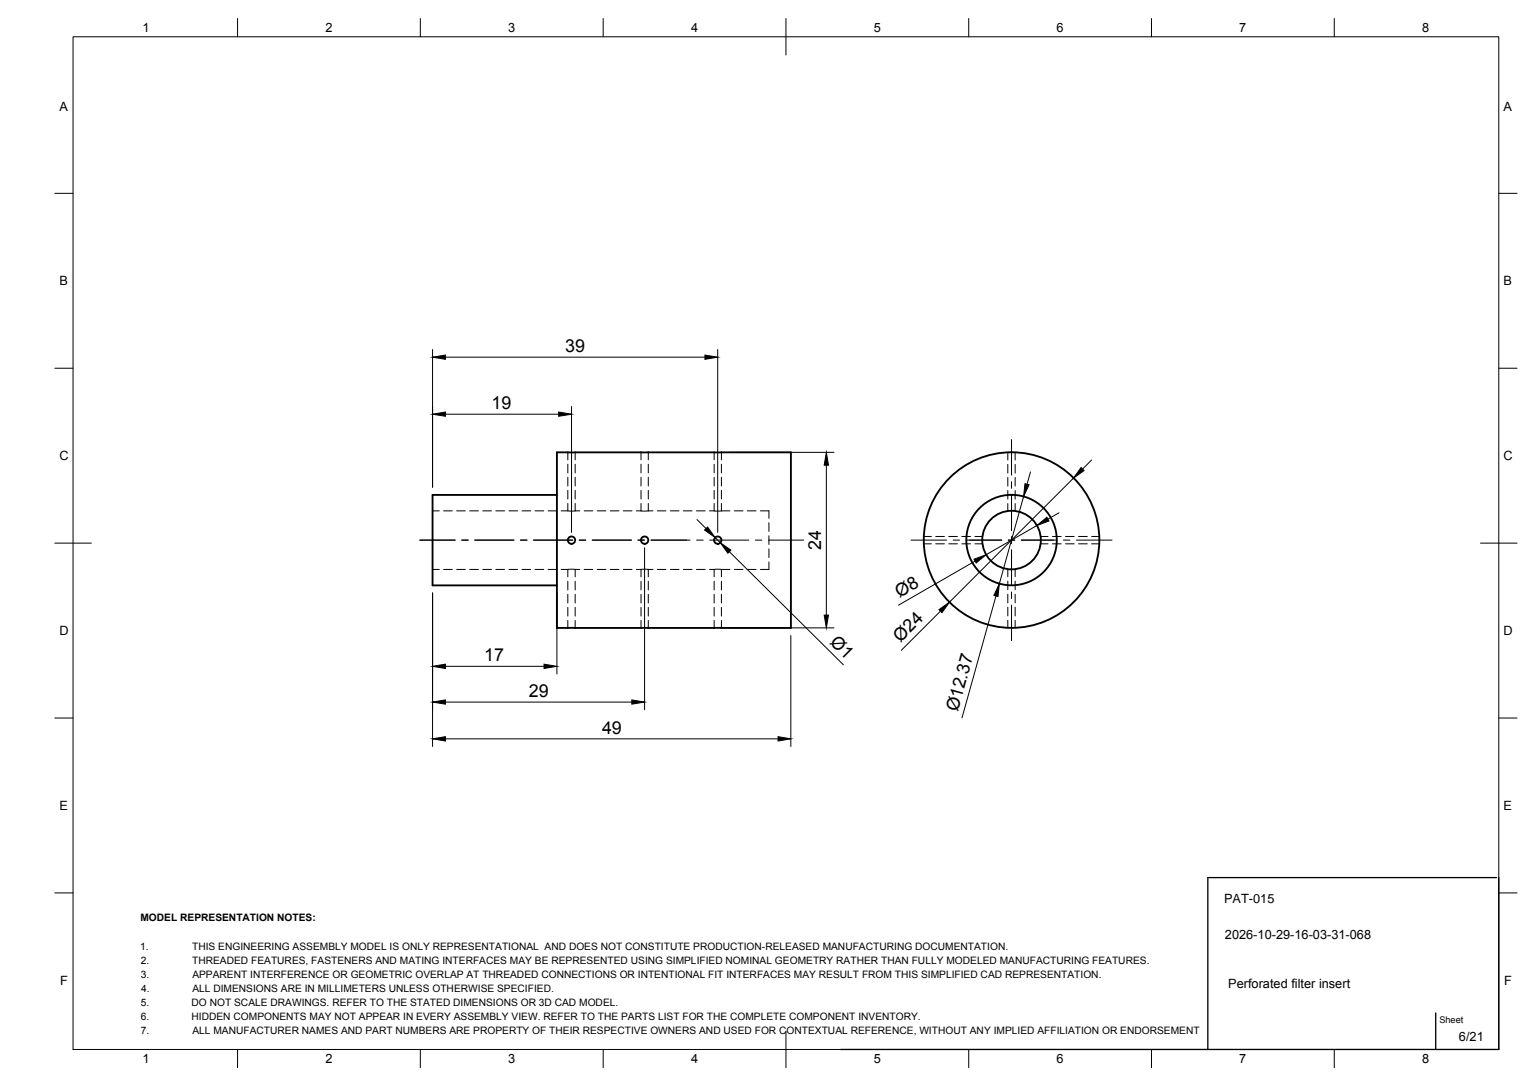
ISO-10303-21;
HEADER;
/* Generated by software containing ST-Developer
 * from STEP Tools, Inc. (www.steptools.com) 
 */

FILE_DESCRIPTION(
/* description */ ('PAT-015'),
/* implementation_level */ '2;1');

FILE_NAME(
/* name */ 'Perforated filter insert.step',
/* time_stamp */ '2026-10-29T16:03:43-07:00',
/* author */ (''),
/* organization */ (''),
/* preprocessor_version */ 'ST-DEVELOPER v20.2',
/* originating_system */ 'Autodesk Translation Framework v15.17.0.0',
/* authorisation */ '');

FILE_SCHEMA (('AUTOMOTIVE_DESIGN { 1 0 10303 214 3 1 1 }'));
ENDSEC;

DATA;
#10=MECHANICAL_DESIGN_GEOMETRIC_PRESENTATION_REPRESENTATION('',(#232),#10266);
#186=SHAPE_REPRESENTATION_RELATIONSHIP('SRR','None',#10357,#209);
#209=ADVANCED_BREP_SHAPE_REPRESENTATION('',(#257),#10245);
#232=STYLED_ITEM('',(#10561),#257);
#257=MANIFOLD_SOLID_BREP('Body1',#4691);
#325=FACE_BOUND('',#967,.T.);
#326=FACE_BOUND('',#968,.T.);
#327=FACE_BOUND('',#969,.T.);
#328=FACE_BOUND('',#970,.T.);
#329=FACE_BOUND('',#971,.T.);
#330=FACE_BOUND('',#972,.T.);
#331=FACE_BOUND('',#973,.T.);
#332=FACE_BOUND('',#974,.T.);
#333=FACE_BOUND('',#975,.T.);
#334=FACE_BOUND('',#979,.T.);
#335=FACE_BOUND('',#981,.T.);
#336=FACE_BOUND('',#982,.T.);
#337=FACE_BOUND('',#983,.T.);
#338=FACE_BOUND('',#984,.T.);
#339=FACE_BOUND('',#985,.T.);
#340=FACE_BOUND('',#986,.T.);
#341=FACE_BOUND('',#987,.T.);
#342=FACE_BOUND('',#988,.T.);
#343=FACE_BOUND('',#989,.T.);
#344=FACE_BOUND('',#991,.T.);
#451=PLANE('',#5134);
#452=PLANE('',#5138);
#453=PLANE('',#5142);
#454=PLANE('',#5143);
#638=FACE_OUTER_BOUND('',#954,.T.);
#639=FACE_OUTER_BOUND('',#955,.T.);
#640=FACE_OUTER_BOUND('',#956,.T.);
#641=FACE_OUTER_BOUND('',#957,.T.);
#642=FACE_OUTER_BOUND('',#958,.T.);
#643=FACE_OUTER_BOUND('',#959,.T.);
#644=FACE_OUTER_BOUND('',#960,.T.);
#645=FACE_OUTER_BOUND('',#961,.T.);
#646=FACE_OUTER_BOUND('',#962,.T.);
#647=FACE_OUTER_BOUND('',#963,.T.);
#648=FACE_OUTER_BOUND('',#964,.T.);
#649=FACE_OUTER_BOUND('',#965,.T.);
#650=FACE_OUTER_BOUND('',#966,.T.);
#651=FACE_OUTER_BOUND('',#976,.T.);
#652=FACE_OUTER_BOUND('',#977,.T.);
#653=FACE_OUTER_BOUND('',#978,.T.);
#654=FACE_OUTER_BOUND('',#980,.T.);
#655=FACE_OUTER_BOUND('',#990,.T.);
#656=FACE_OUTER_BOUND('',#992,.T.);
#954=EDGE_LOOP('',(#3367,#3368,#3369,#3370));
#955=EDGE_LOOP('',(#3371,#3372,#3373,#3374));
#956=EDGE_LOOP('',(#3375,#3376,#3377,#3378));
#957=EDGE_LOOP('',(#3379,#3380,#3381,#3382));
#958=EDGE_LOOP('',(#3383,#3384,#3385,#3386));
#959=EDGE_LOOP('',(#3387,#3388,#3389,#3390));
#960=EDGE_LOOP('',(#3391,#3392,#3393,#3394,#3395,#3396,#3397,#3398));
#961=EDGE_LOOP('',(#3399,#3400,#3401,#3402,#3403,#3404));
#962=EDGE_LOOP('',(#3405,#3406,#3407,#3408,#3409,#3410,#3411,#3412));
#963=EDGE_LOOP('',(#3413,#3414,#3415,#3416,#3417,#3418));
#964=EDGE_LOOP('',(#3419,#3420,#3421,#3422,#3423,#3424,#3425,#3426));
#965=EDGE_LOOP('',(#3427,#3428,#3429,#3430,#3431,#3432));
#966=EDGE_LOOP('',(#3433,#3434,#3435,#3436,#3437,#3438,#3439,#3440,#3441,
#3442,#3443,#3444,#3445,#3446,#3447,#3448,#3449,#3450,#3451));
#967=EDGE_LOOP('',(#3452));
#968=EDGE_LOOP('',(#3453));
#969=EDGE_LOOP('',(#3454));
#970=EDGE_LOOP('',(#3455));
#971=EDGE_LOOP('',(#3456));
#972=EDGE_LOOP('',(#3457));
#973=EDGE_LOOP('',(#3458,#3459));
#974=EDGE_LOOP('',(#3460,#3461));
#975=EDGE_LOOP('',(#3462,#3463));
#976=EDGE_LOOP('',(#3464));
#977=EDGE_LOOP('',(#3465,#3466,#3467,#3468));
#978=EDGE_LOOP('',(#3469));
#979=EDGE_LOOP('',(#3470));
#980=EDGE_LOOP('',(#3471,#3472,#3473,#3474,#3475,#3476,#3477,#3478,#3479,
#3480,#3481,#3482,#3483,#3484,#3485,#3486,#3487,#3488,#3489));
#981=EDGE_LOOP('',(#3490));
#982=EDGE_LOOP('',(#3491));
#983=EDGE_LOOP('',(#3492));
#984=EDGE_LOOP('',(#3493));
#985=EDGE_LOOP('',(#3494));
#986=EDGE_LOOP('',(#3495));
#987=EDGE_LOOP('',(#3496,#3497));
#988=EDGE_LOOP('',(#3498,#3499));
#989=EDGE_LOOP('',(#3500,#3501));
#990=EDGE_LOOP('',(#3502));
#991=EDGE_LOOP('',(#3503));
#992=EDGE_LOOP('',(#3504));
#1277=B_SPLINE_CURVE_WITH_KNOTS('',3,(#7517,#7518,#7519,#7520,#7521,#7522,
#7523,#7524,#7525,#7526,#7527,#7528,#7529,#7530,#7531,#7532,#7533,#7534,
#7535,#7536,#7537,#7538,#7539,#7540,#7541,#7542,#7543,#7544,#7545,#7546,
#7547,#7548,#7549,#7550),.UNSPECIFIED.,.T.,.F.,(4,2,2,2,2,2,2,2,2,2,2,2,
2,2,2,2,4),(0.,0.0188366744349197,0.0376733488698393,0.0565100213871705,
0.0753466939045016,0.0941833664218328,0.113020038939164,0.131856713374084,
0.150693387809003,0.169530062243923,0.188366736678843,0.207203409196174,
0.226040081713505,0.244876754230836,0.263713426748167,0.282550101183087,
0.301386775618006),.UNSPECIFIED.);
#1278=B_SPLINE_CURVE_WITH_KNOTS('',3,(#7553,#7554,#7555,#7556,#7557,#7558,
#7559,#7560,#7561,#7562,#7563,#7564,#7565,#7566,#7567,#7568,#7569,#7570,
#7571,#7572,#7573,#7574,#7575,#7576,#7577,#7578,#7579,#7580,#7581,#7582,
#7583,#7584,#7585,#7586),.UNSPECIFIED.,.T.,.F.,(4,2,2,2,2,2,2,2,2,2,2,2,
2,2,2,2,4),(0.,0.0188556028927646,0.0377112057855292,0.0565666511569687,
0.0754220965284081,0.0942775418998475,0.113132987271287,0.131988590164052,
0.150844193056816,0.169699795949581,0.188555398842345,0.207410844213785,
0.226266289585224,0.245121734956664,0.263977180328103,0.282832783220868,
0.301688386113632),.UNSPECIFIED.);
#1279=B_SPLINE_CURVE_WITH_KNOTS('',3,(#7589,#7590,#7591,#7592,#7593,#7594,
#7595,#7596,#7597,#7598,#7599,#7600,#7601,#7602,#7603,#7604,#7605,#7606,
#7607,#7608,#7609,#7610,#7611,#7612,#7613,#7614,#7615,#7616,#7617,#7618,
#7619,#7620,#7621,#7622),.UNSPECIFIED.,.T.,.F.,(4,2,2,2,2,2,2,2,2,2,2,2,
2,2,2,2,4),(0.,0.0188556028927646,0.0377112057855292,0.0565666511569687,
0.0754220965284081,0.0942775418998475,0.113132987271287,0.131988590164052,
0.150844193056816,0.169699795949581,0.188555398842345,0.207410844213785,
0.226266289585224,0.245121734956664,0.263977180328103,0.282832783220868,
0.301688386113632),.UNSPECIFIED.);
#1280=B_SPLINE_CURVE_WITH_KNOTS('',3,(#7625,#7626,#7627,#7628,#7629,#7630,
#7631,#7632,#7633,#7634,#7635,#7636,#7637,#7638,#7639,#7640,#7641,#7642,
#7643,#7644,#7645,#7646,#7647,#7648,#7649,#7650,#7651,#7652,#7653,#7654,
#7655,#7656,#7657,#7658),.UNSPECIFIED.,.T.,.F.,(4,2,2,2,2,2,2,2,2,2,2,2,
2,2,2,2,4),(0.,0.0188366744349197,0.0376733488698393,0.0565100213871705,
0.0753466939045016,0.0941833664218328,0.113020038939164,0.131856713374084,
0.150693387809003,0.169530062243923,0.188366736678843,0.207203409196174,
0.226040081713505,0.244876754230836,0.263713426748167,0.282550101183087,
0.301386775618006),.UNSPECIFIED.);
#1281=B_SPLINE_CURVE_WITH_KNOTS('',3,(#7661,#7662,#7663,#7664,#7665,#7666,
#7667,#7668,#7669,#7670,#7671,#7672,#7673,#7674,#7675,#7676,#7677,#7678,
#7679,#7680,#7681,#7682,#7683,#7684,#7685,#7686,#7687,#7688,#7689,#7690,
#7691,#7692,#7693,#7694),.UNSPECIFIED.,.T.,.F.,(4,2,2,2,2,2,2,2,2,2,2,2,
2,2,2,2,4),(0.,0.0188366744349197,0.0376733488698393,0.0565100213871705,
0.0753466939045016,0.0941833664218328,0.113020038939164,0.131856713374084,
0.150693387809003,0.169530062243923,0.188366736678843,0.207203409196174,
0.226040081713505,0.244876754230836,0.263713426748167,0.282550101183087,
0.301386775618007),.UNSPECIFIED.);
#1282=B_SPLINE_CURVE_WITH_KNOTS('',3,(#7697,#7698,#7699,#7700,#7701,#7702,
#7703,#7704,#7705,#7706,#7707,#7708,#7709,#7710,#7711,#7712,#7713,#7714,
#7715,#7716,#7717,#7718,#7719,#7720,#7721,#7722,#7723,#7724,#7725,#7726,
#7727,#7728,#7729,#7730),.UNSPECIFIED.,.T.,.F.,(4,2,2,2,2,2,2,2,2,2,2,2,
2,2,2,2,4),(0.,0.0188556028927646,0.0377112057855293,0.0565666511569687,
0.0754220965284081,0.0942775418998476,0.113132987271287,0.131988590164052,
0.150844193056816,0.169699795949581,0.188555398842346,0.207410844213785,
0.226266289585224,0.245121734956664,0.263977180328103,0.282832783220868,
0.301688386113632),.UNSPECIFIED.);
#1283=B_SPLINE_CURVE_WITH_KNOTS('',3,(#7733,#7734,#7735,#7736,#7737,#7738,
#7739,#7740,#7741,#7742,#7743,#7744,#7745,#7746,#7747,#7748,#7749,#7750,
#7751,#7752,#7753,#7754,#7755,#7756,#7757,#7758,#7759,#7760,#7761,#7762,
#7763,#7764,#7765,#7766),.UNSPECIFIED.,.T.,.F.,(4,2,2,2,2,2,2,2,2,2,2,2,
2,2,2,2,4),(0.,0.0188556028927646,0.0377112057855292,0.0565666511569687,
0.0754220965284081,0.0942775418998475,0.113132987271287,0.131988590164052,
0.150844193056816,0.169699795949581,0.188555398842345,0.207410844213785,
0.226266289585224,0.245121734956664,0.263977180328103,0.282832783220868,
0.301688386113632),.UNSPECIFIED.);
#1284=B_SPLINE_CURVE_WITH_KNOTS('',3,(#7769,#7770,#7771,#7772,#7773,#7774,
#7775,#7776,#7777,#7778,#7779,#7780,#7781,#7782,#7783,#7784,#7785,#7786,
#7787,#7788,#7789,#7790,#7791,#7792,#7793,#7794,#7795,#7796,#7797,#7798,
#7799,#7800,#7801,#7802),.UNSPECIFIED.,.T.,.F.,(4,2,2,2,2,2,2,2,2,2,2,2,
2,2,2,2,4),(0.,0.0188366744349198,0.0376733488698396,0.0565100213871707,
0.0753466939045018,0.094183366421833,0.113020038939164,0.131856713374084,
0.150693387809003,0.169530062243923,0.188366736678843,0.207203409196174,
0.226040081713505,0.244876754230836,0.263713426748167,0.282550101183087,
0.301386775618007),.UNSPECIFIED.);
#1285=B_SPLINE_CURVE_WITH_KNOTS('',3,(#7805,#7806,#7807,#7808,#7809,#7810,
#7811,#7812,#7813,#7814,#7815,#7816,#7817,#7818,#7819,#7820,#7821,#7822,
#7823,#7824,#7825,#7826,#7827,#7828,#7829,#7830,#7831,#7832,#7833,#7834,
#7835,#7836,#7837,#7838),.UNSPECIFIED.,.T.,.F.,(4,2,2,2,2,2,2,2,2,2,2,2,
2,2,2,2,4),(0.,0.0188366744349197,0.0376733488698393,0.0565100213871705,
0.0753466939045016,0.0941833664218328,0.113020038939164,0.131856713374084,
0.150693387809003,0.169530062243923,0.188366736678842,0.207203409196173,
0.226040081713505,0.244876754230836,0.263713426748167,0.282550101183086,
0.301386775618006),.UNSPECIFIED.);
#1286=B_SPLINE_CURVE_WITH_KNOTS('',3,(#7841,#7842,#7843,#7844,#7845,#7846,
#7847,#7848,#7849,#7850,#7851,#7852,#7853,#7854,#7855,#7856,#7857,#7858,
#7859,#7860,#7861,#7862,#7863,#7864,#7865,#7866,#7867,#7868,#7869,#7870,
#7871,#7872,#7873,#7874),.UNSPECIFIED.,.T.,.F.,(4,2,2,2,2,2,2,2,2,2,2,2,
2,2,2,2,4),(0.,0.0188556028927646,0.0377112057855292,0.0565666511569687,
0.0754220965284081,0.0942775418998475,0.113132987271287,0.131988590164052,
0.150844193056816,0.169699795949581,0.188555398842345,0.207410844213785,
0.226266289585224,0.245121734956664,0.263977180328103,0.282832783220868,
0.301688386113632),.UNSPECIFIED.);
#1287=B_SPLINE_CURVE_WITH_KNOTS('',3,(#7877,#7878,#7879,#7880,#7881,#7882,
#7883,#7884,#7885,#7886,#7887,#7888,#7889,#7890,#7891,#7892,#7893,#7894,
#7895,#7896,#7897,#7898,#7899,#7900,#7901,#7902,#7903,#7904,#7905,#7906,
#7907,#7908,#7909,#7910),.UNSPECIFIED.,.T.,.F.,(4,2,2,2,2,2,2,2,2,2,2,2,
2,2,2,2,4),(0.,0.0188556028927646,0.0377112057855292,0.0565666511569687,
0.0754220965284081,0.0942775418998475,0.113132987271287,0.131988590164052,
0.150844193056816,0.169699795949581,0.188555398842345,0.207410844213785,
0.226266289585224,0.245121734956664,0.263977180328103,0.282832783220868,
0.301688386113632),.UNSPECIFIED.);
#1288=B_SPLINE_CURVE_WITH_KNOTS('',3,(#7913,#7914,#7915,#7916,#7917,#7918,
#7919,#7920,#7921,#7922,#7923,#7924,#7925,#7926,#7927,#7928,#7929,#7930,
#7931,#7932,#7933,#7934,#7935,#7936,#7937,#7938,#7939,#7940,#7941,#7942,
#7943,#7944,#7945,#7946),.UNSPECIFIED.,.T.,.F.,(4,2,2,2,2,2,2,2,2,2,2,2,
2,2,2,2,4),(0.,0.0188366744349194,0.0376733488698389,0.0565100213871701,
0.0753466939045014,0.0941833664218326,0.113020038939164,0.131856713374083,
0.150693387809003,0.169530062243922,0.188366736678842,0.207203409196173,
0.226040081713504,0.244876754230835,0.263713426748167,0.282550101183086,
0.301386775618006),.UNSPECIFIED.);
#1289=B_SPLINE_CURVE_WITH_KNOTS('',3,(#7950,#7951,#7952,#7953,#7954,#7955,
#7956,#7957,#7958,#7959),.UNSPECIFIED.,.F.,.F.,(4,2,2,2,4),(0.,0.0188366744349197,
0.0376733488698393,0.0565100213871704,0.0753466939045014),.UNSPECIFIED.);
#1290=B_SPLINE_CURVE_WITH_KNOTS('',3,(#7961,#7962,#7963,#7964,#7965,#7966,
#7967,#7968,#7969,#7970),.UNSPECIFIED.,.F.,.F.,(4,2,2,2,4),(0.226040081713504,
0.244876754230835,0.263713426748166,0.282550101183086,0.301386775618006),
 .UNSPECIFIED.);
#1291=B_SPLINE_CURVE_WITH_KNOTS('',3,(#7971,#7972,#7973,#7974,#7975,#7976,
#7977,#7978,#7979,#7980,#7981,#7982,#7983,#7984,#7985,#7986,#7987,#7988),
 .UNSPECIFIED.,.F.,.F.,(4,2,2,2,2,2,2,2,4),(0.0753466939045014,0.0941833664218325,
0.113020038939164,0.131856713374083,0.150693387809003,0.169530062243923,
0.188366736678842,0.207203409196173,0.226040081713504),.UNSPECIFIED.);
#1292=B_SPLINE_CURVE_WITH_KNOTS('',3,(#7992,#7993,#7994,#7995,#7996,#7997,
#7998,#7999,#8000,#8001,#8002,#8003,#8004,#8005,#8006,#8007,#8008,#8009),
 .UNSPECIFIED.,.F.,.F.,(4,2,2,2,2,2,2,2,4),(0.0754220965284079,0.0942775418998473,
0.113132987271287,0.131988590164051,0.150844193056816,0.16969979594958,
0.188555398842345,0.207410844213784,0.226266289585224),.UNSPECIFIED.);
#1293=B_SPLINE_CURVE_WITH_KNOTS('',3,(#8011,#8012,#8013,#8014,#8015,#8016,
#8017,#8018,#8019,#8020),.UNSPECIFIED.,.F.,.F.,(4,2,2,2,4),(0.,0.0188556028927646,
0.0377112057855293,0.0565666511569686,0.0754220965284079),.UNSPECIFIED.);
#1294=B_SPLINE_CURVE_WITH_KNOTS('',3,(#8021,#8022,#8023,#8024,#8025,#8026,
#8027,#8028,#8029,#8030),.UNSPECIFIED.,.F.,.F.,(4,2,2,2,4),(0.226266289585224,
0.245121734956663,0.263977180328102,0.282832783220867,0.301688386113632),
 .UNSPECIFIED.);
#1295=B_SPLINE_CURVE_WITH_KNOTS('',3,(#8034,#8035,#8036,#8037,#8038,#8039,
#8040,#8041,#8042,#8043),.UNSPECIFIED.,.F.,.F.,(4,2,2,2,4),(0.,0.0188556028927646,
0.0377112057855293,0.0565666511569686,0.0754220965284079),.UNSPECIFIED.);
#1296=B_SPLINE_CURVE_WITH_KNOTS('',3,(#8044,#8045,#8046,#8047,#8048,#8049,
#8050,#8051,#8052,#8053,#8054,#8055,#8056,#8057,#8058,#8059,#8060,#8061,
#8062,#8063,#8064,#8065,#8066,#8067,#8068,#8069),.UNSPECIFIED.,.F.,.F.,
(4,2,2,2,2,2,2,2,2,2,2,2,4),(0.0754220965284079,0.0942775418998473,0.113132987271287,
0.131988590164051,0.150844193056816,0.16969979594958,0.188555398842345,
0.207410844213784,0.226266289585224,0.245121734956663,0.263977180328102,
0.282832783220867,0.301688386113632),.UNSPECIFIED.);
#1297=B_SPLINE_CURVE_WITH_KNOTS('',3,(#8073,#8074,#8075,#8076,#8077,#8078,
#8079,#8080,#8081,#8082,#8083,#8084,#8085,#8086,#8087,#8088,#8089,#8090,
#8091,#8092,#8093,#8094,#8095,#8096,#8097,#8098),.UNSPECIFIED.,.F.,.F.,
(4,2,2,2,2,2,2,2,2,2,2,2,4),(0.,0.0188366744349197,0.0376733488698393,0.0565100213871704,
0.0753466939045015,0.0941833664218325,0.113020038939164,0.131856713374083,
0.150693387809003,0.169530062243923,0.188366736678842,0.207203409196173,
0.226040081713504),.UNSPECIFIED.);
#1298=B_SPLINE_CURVE_WITH_KNOTS('',3,(#8099,#8100,#8101,#8102,#8103,#8104,
#8105,#8106,#8107,#8108),.UNSPECIFIED.,.F.,.F.,(4,2,2,2,4),(0.226040081713504,
0.244876754230835,0.263713426748167,0.282550101183086,0.301386775618006),
 .UNSPECIFIED.);
#1299=B_SPLINE_CURVE_WITH_KNOTS('',3,(#8112,#8113,#8114,#8115,#8116,#8117,
#8118,#8119,#8120,#8121),.UNSPECIFIED.,.F.,.F.,(4,2,2,2,4),(0.,0.0188366744349197,
0.0376733488698393,0.0565100213871705,0.0753466939045016),.UNSPECIFIED.);
#1300=B_SPLINE_CURVE_WITH_KNOTS('',3,(#8123,#8124,#8125,#8126,#8127,#8128,
#8129,#8130,#8131,#8132),.UNSPECIFIED.,.F.,.F.,(4,2,2,2,4),(0.226040081713505,
0.244876754230836,0.263713426748167,0.282550101183087,0.301386775618007),
 .UNSPECIFIED.);
#1301=B_SPLINE_CURVE_WITH_KNOTS('',3,(#8133,#8134,#8135,#8136,#8137,#8138,
#8139,#8140,#8141,#8142,#8143,#8144,#8145,#8146,#8147,#8148,#8149,#8150),
 .UNSPECIFIED.,.F.,.F.,(4,2,2,2,2,2,2,2,4),(0.0753466939045016,0.0941833664218328,
0.113020038939164,0.131856713374084,0.150693387809003,0.169530062243923,
0.188366736678843,0.207203409196174,0.226040081713505),.UNSPECIFIED.);
#1302=B_SPLINE_CURVE_WITH_KNOTS('',3,(#8154,#8155,#8156,#8157,#8158,#8159,
#8160,#8161,#8162,#8163,#8164,#8165,#8166,#8167,#8168,#8169,#8170,#8171),
 .UNSPECIFIED.,.F.,.F.,(4,2,2,2,2,2,2,2,4),(0.0754220965284082,0.0942775418998476,
0.113132987271287,0.131988590164052,0.150844193056816,0.169699795949581,
0.188555398842346,0.207410844213785,0.226266289585224),.UNSPECIFIED.);
#1303=B_SPLINE_CURVE_WITH_KNOTS('',3,(#8173,#8174,#8175,#8176,#8177,#8178,
#8179,#8180,#8181,#8182),.UNSPECIFIED.,.F.,.F.,(4,2,2,2,4),(0.,0.0188556028927646,
0.0377112057855293,0.0565666511569687,0.0754220965284082),.UNSPECIFIED.);
#1304=B_SPLINE_CURVE_WITH_KNOTS('',3,(#8183,#8184,#8185,#8186,#8187,#8188,
#8189,#8190,#8191,#8192),.UNSPECIFIED.,.F.,.F.,(4,2,2,2,4),(0.226266289585224,
0.245121734956664,0.263977180328103,0.282832783220868,0.301688386113633),
 .UNSPECIFIED.);
#1305=B_SPLINE_CURVE_WITH_KNOTS('',3,(#8196,#8197,#8198,#8199,#8200,#8201,
#8202,#8203,#8204,#8205),.UNSPECIFIED.,.F.,.F.,(4,2,2,2,4),(0.,0.0188556028927646,
0.0377112057855293,0.0565666511569687,0.0754220965284081),.UNSPECIFIED.);
#1306=B_SPLINE_CURVE_WITH_KNOTS('',3,(#8206,#8207,#8208,#8209,#8210,#8211,
#8212,#8213,#8214,#8215,#8216,#8217,#8218,#8219,#8220,#8221,#8222,#8223,
#8224,#8225,#8226,#8227,#8228,#8229,#8230,#8231),.UNSPECIFIED.,.F.,.F.,
(4,2,2,2,2,2,2,2,2,2,2,2,4),(0.0754220965284081,0.0942775418998476,0.113132987271287,
0.131988590164052,0.150844193056816,0.169699795949581,0.188555398842346,
0.207410844213785,0.226266289585224,0.245121734956664,0.263977180328103,
0.282832783220868,0.301688386113633),.UNSPECIFIED.);
#1307=B_SPLINE_CURVE_WITH_KNOTS('',3,(#8235,#8236,#8237,#8238,#8239,#8240,
#8241,#8242,#8243,#8244,#8245,#8246,#8247,#8248,#8249,#8250,#8251,#8252,
#8253,#8254,#8255,#8256,#8257,#8258,#8259,#8260),.UNSPECIFIED.,.F.,.F.,
(4,2,2,2,2,2,2,2,2,2,2,2,4),(0.,0.0188366744349197,0.0376733488698393,0.0565100213871705,
0.0753466939045017,0.0941833664218329,0.113020038939164,0.131856713374084,
0.150693387809003,0.169530062243923,0.188366736678843,0.207203409196174,
0.226040081713505),.UNSPECIFIED.);
#1308=B_SPLINE_CURVE_WITH_KNOTS('',3,(#8261,#8262,#8263,#8264,#8265,#8266,
#8267,#8268,#8269,#8270),.UNSPECIFIED.,.F.,.F.,(4,2,2,2,4),(0.226040081713505,
0.244876754230836,0.263713426748167,0.282550101183087,0.301386775618007),
 .UNSPECIFIED.);
#1309=B_SPLINE_CURVE_WITH_KNOTS('',3,(#8274,#8275,#8276,#8277,#8278,#8279,
#8280,#8281,#8282,#8283),.UNSPECIFIED.,.F.,.F.,(4,2,2,2,4),(0.,0.0188366744349197,
0.0376733488698393,0.0565100213871705,0.0753466939045016),.UNSPECIFIED.);
#1310=B_SPLINE_CURVE_WITH_KNOTS('',3,(#8285,#8286,#8287,#8288,#8289,#8290,
#8291,#8292,#8293,#8294),.UNSPECIFIED.,.F.,.F.,(4,2,2,2,4),(0.226040081713505,
0.244876754230836,0.263713426748167,0.282550101183087,0.301386775618006),
 .UNSPECIFIED.);
#1311=B_SPLINE_CURVE_WITH_KNOTS('',3,(#8295,#8296,#8297,#8298,#8299,#8300,
#8301,#8302,#8303,#8304,#8305,#8306,#8307,#8308,#8309,#8310,#8311,#8312),
 .UNSPECIFIED.,.F.,.F.,(4,2,2,2,2,2,2,2,4),(0.0753466939045016,0.0941833664218328,
0.113020038939164,0.131856713374084,0.150693387809003,0.169530062243923,
0.188366736678842,0.207203409196173,0.226040081713505),.UNSPECIFIED.);
#1312=B_SPLINE_CURVE_WITH_KNOTS('',3,(#8316,#8317,#8318,#8319,#8320,#8321,
#8322,#8323,#8324,#8325,#8326,#8327,#8328,#8329,#8330,#8331,#8332,#8333),
 .UNSPECIFIED.,.F.,.F.,(4,2,2,2,2,2,2,2,4),(0.0754220965284081,0.0942775418998475,
0.113132987271287,0.131988590164052,0.150844193056816,0.169699795949581,
0.188555398842345,0.207410844213785,0.226266289585224),.UNSPECIFIED.);
#1313=B_SPLINE_CURVE_WITH_KNOTS('',3,(#8335,#8336,#8337,#8338,#8339,#8340,
#8341,#8342,#8343,#8344),.UNSPECIFIED.,.F.,.F.,(4,2,2,2,4),(0.,0.0188556028927646,
0.0377112057855293,0.0565666511569687,0.0754220965284081),.UNSPECIFIED.);
#1314=B_SPLINE_CURVE_WITH_KNOTS('',3,(#8345,#8346,#8347,#8348,#8349,#8350,
#8351,#8352,#8353,#8354),.UNSPECIFIED.,.F.,.F.,(4,2,2,2,4),(0.226266289585224,
0.245121734956664,0.263977180328103,0.282832783220868,0.301688386113632),
 .UNSPECIFIED.);
#1315=B_SPLINE_CURVE_WITH_KNOTS('',3,(#8358,#8359,#8360,#8361,#8362,#8363,
#8364,#8365,#8366,#8367),.UNSPECIFIED.,.F.,.F.,(4,2,2,2,4),(0.,0.0188556028927646,
0.0377112057855293,0.0565666511569687,0.0754220965284081),.UNSPECIFIED.);
#1316=B_SPLINE_CURVE_WITH_KNOTS('',3,(#8368,#8369,#8370,#8371,#8372,#8373,
#8374,#8375,#8376,#8377,#8378,#8379,#8380,#8381,#8382,#8383,#8384,#8385,
#8386,#8387,#8388,#8389,#8390,#8391,#8392,#8393),.UNSPECIFIED.,.F.,.F.,
(4,2,2,2,2,2,2,2,2,2,2,2,4),(0.0754220965284081,0.0942775418998476,0.113132987271287,
0.131988590164052,0.150844193056816,0.169699795949581,0.188555398842345,
0.207410844213785,0.226266289585224,0.245121734956664,0.263977180328103,
0.282832783220868,0.301688386113632),.UNSPECIFIED.);
#1317=B_SPLINE_CURVE_WITH_KNOTS('',3,(#8397,#8398,#8399,#8400,#8401,#8402,
#8403,#8404,#8405,#8406,#8407,#8408,#8409,#8410,#8411,#8412,#8413,#8414,
#8415,#8416,#8417,#8418,#8419,#8420,#8421,#8422),.UNSPECIFIED.,.F.,.F.,
(4,2,2,2,2,2,2,2,2,2,2,2,4),(0.,0.0188366744349194,0.0376733488698389,0.0565100213871702,
0.0753466939045014,0.0941833664218327,0.113020038939164,0.131856713374083,
0.150693387809003,0.169530062243922,0.188366736678842,0.207203409196173,
0.226040081713504),.UNSPECIFIED.);
#1318=B_SPLINE_CURVE_WITH_KNOTS('',3,(#8423,#8424,#8425,#8426,#8427,#8428,
#8429,#8430,#8431,#8432),.UNSPECIFIED.,.F.,.F.,(4,2,2,2,4),(0.226040081713504,
0.244876754230836,0.263713426748167,0.282550101183086,0.301386775618006),
 .UNSPECIFIED.);
#1366=LINE('',#7552,#1646);
#1367=LINE('',#7624,#1647);
#1368=LINE('',#7696,#1648);
#1369=LINE('',#7768,#1649);
#1370=LINE('',#7840,#1650);
#1371=LINE('',#7912,#1651);
#1372=LINE('',#7990,#1652);
#1373=LINE('',#8071,#1653);
#1374=LINE('',#8152,#1654);
#1375=LINE('',#8233,#1655);
#1376=LINE('',#8314,#1656);
#1377=LINE('',#8395,#1657);
#1378=LINE('',#8436,#1658);
#1379=LINE('',#8437,#1659);
#1380=LINE('',#8438,#1660);
#1381=LINE('',#8440,#1661);
#1382=LINE('',#8447,#1662);
#1383=LINE('',#8453,#1663);
#1384=LINE('',#8454,#1664);
#1385=LINE('',#8455,#1665);
#1386=LINE('',#8457,#1666);
#1646=VECTOR('',#5899,0.05);
#1647=VECTOR('',#5902,0.05);
#1648=VECTOR('',#5905,0.05);
#1649=VECTOR('',#5908,0.05);
#1650=VECTOR('',#5911,0.05);
#1651=VECTOR('',#5914,0.05);
#1652=VECTOR('',#5917,0.0499999999999998);
#1653=VECTOR('',#5920,0.0499999999999998);
#1654=VECTOR('',#5923,0.05);
#1655=VECTOR('',#5926,0.05);
#1656=VECTOR('',#5929,0.05);
#1657=VECTOR('',#5932,0.05);
#1658=VECTOR('',#5937,0.4);
#1659=VECTOR('',#5938,0.4);
#1660=VECTOR('',#5939,0.4);
#1661=VECTOR('',#5940,0.4);
#1662=VECTOR('',#5949,0.6185);
#1663=VECTOR('',#5958,1.2);
#1664=VECTOR('',#5959,1.2);
#1665=VECTOR('',#5960,1.2);
#1666=VECTOR('',#5961,1.2);
#1947=CIRCLE('',#5132,0.4);
#1948=CIRCLE('',#5133,0.4);
#1949=CIRCLE('',#5136,0.6185);
#1950=CIRCLE('',#5137,0.6185);
#1951=CIRCLE('',#5140,1.2);
#1952=CIRCLE('',#5141,1.2);
#2201=VERTEX_POINT('',#7516);
#2202=VERTEX_POINT('',#7551);
#2203=VERTEX_POINT('',#7588);
#2204=VERTEX_POINT('',#7623);
#2205=VERTEX_POINT('',#7660);
#2206=VERTEX_POINT('',#7695);
#2207=VERTEX_POINT('',#7732);
#2208=VERTEX_POINT('',#7767);
#2209=VERTEX_POINT('',#7804);
#2210=VERTEX_POINT('',#7839);
#2211=VERTEX_POINT('',#7876);
#2212=VERTEX_POINT('',#7911);
#2213=VERTEX_POINT('',#7948);
#2214=VERTEX_POINT('',#7949);
#2215=VERTEX_POINT('',#7960);
#2216=VERTEX_POINT('',#7989);
#2217=VERTEX_POINT('',#7991);
#2218=VERTEX_POINT('',#8010);
#2219=VERTEX_POINT('',#8032);
#2220=VERTEX_POINT('',#8033);
#2221=VERTEX_POINT('',#8070);
#2222=VERTEX_POINT('',#8072);
#2223=VERTEX_POINT('',#8110);
#2224=VERTEX_POINT('',#8111);
#2225=VERTEX_POINT('',#8122);
#2226=VERTEX_POINT('',#8151);
#2227=VERTEX_POINT('',#8153);
#2228=VERTEX_POINT('',#8172);
#2229=VERTEX_POINT('',#8194);
#2230=VERTEX_POINT('',#8195);
#2231=VERTEX_POINT('',#8232);
#2232=VERTEX_POINT('',#8234);
#2233=VERTEX_POINT('',#8272);
#2234=VERTEX_POINT('',#8273);
#2235=VERTEX_POINT('',#8284);
#2236=VERTEX_POINT('',#8313);
#2237=VERTEX_POINT('',#8315);
#2238=VERTEX_POINT('',#8334);
#2239=VERTEX_POINT('',#8356);
#2240=VERTEX_POINT('',#8357);
#2241=VERTEX_POINT('',#8394);
#2242=VERTEX_POINT('',#8396);
#2243=VERTEX_POINT('',#8434);
#2244=VERTEX_POINT('',#8439);
#2245=VERTEX_POINT('',#8444);
#2246=VERTEX_POINT('',#8446);
#2247=VERTEX_POINT('',#8451);
#2248=VERTEX_POINT('',#8456);
#2639=EDGE_CURVE('',#2201,#2201,#1277,.T.);
#2640=EDGE_CURVE('',#2201,#2202,#1366,.T.);
#2641=EDGE_CURVE('',#2202,#2202,#1278,.T.);
#2642=EDGE_CURVE('',#2203,#2203,#1279,.T.);
#2643=EDGE_CURVE('',#2203,#2204,#1367,.T.);
#2644=EDGE_CURVE('',#2204,#2204,#1280,.T.);
#2645=EDGE_CURVE('',#2205,#2205,#1281,.T.);
#2646=EDGE_CURVE('',#2205,#2206,#1368,.T.);
#2647=EDGE_CURVE('',#2206,#2206,#1282,.T.);
#2648=EDGE_CURVE('',#2207,#2207,#1283,.T.);
#2649=EDGE_CURVE('',#2207,#2208,#1369,.T.);
#2650=EDGE_CURVE('',#2208,#2208,#1284,.T.);
#2651=EDGE_CURVE('',#2209,#2209,#1285,.T.);
#2652=EDGE_CURVE('',#2209,#2210,#1370,.T.);
#2653=EDGE_CURVE('',#2210,#2210,#1286,.T.);
#2654=EDGE_CURVE('',#2211,#2211,#1287,.T.);
#2655=EDGE_CURVE('',#2211,#2212,#1371,.T.);
#2656=EDGE_CURVE('',#2212,#2212,#1288,.T.);
#2657=EDGE_CURVE('',#2213,#2214,#1289,.T.);
#2658=EDGE_CURVE('',#2215,#2213,#1290,.T.);
#2659=EDGE_CURVE('',#2214,#2215,#1291,.T.);
#2660=EDGE_CURVE('',#2214,#2216,#1372,.T.);
#2661=EDGE_CURVE('',#2217,#2216,#1292,.T.);
#2662=EDGE_CURVE('',#2218,#2217,#1293,.T.);
#2663=EDGE_CURVE('',#2216,#2218,#1294,.T.);
#2664=EDGE_CURVE('',#2219,#2220,#1295,.T.);
#2665=EDGE_CURVE('',#2220,#2219,#1296,.T.);
#2666=EDGE_CURVE('',#2220,#2221,#1373,.T.);
#2667=EDGE_CURVE('',#2222,#2221,#1297,.T.);
#2668=EDGE_CURVE('',#2221,#2222,#1298,.T.);
#2669=EDGE_CURVE('',#2223,#2224,#1299,.T.);
#2670=EDGE_CURVE('',#2225,#2223,#1300,.T.);
#2671=EDGE_CURVE('',#2224,#2225,#1301,.T.);
#2672=EDGE_CURVE('',#2224,#2226,#1374,.T.);
#2673=EDGE_CURVE('',#2227,#2226,#1302,.T.);
#2674=EDGE_CURVE('',#2228,#2227,#1303,.T.);
#2675=EDGE_CURVE('',#2226,#2228,#1304,.T.);
#2676=EDGE_CURVE('',#2229,#2230,#1305,.T.);
#2677=EDGE_CURVE('',#2230,#2229,#1306,.T.);
#2678=EDGE_CURVE('',#2230,#2231,#1375,.T.);
#2679=EDGE_CURVE('',#2232,#2231,#1307,.T.);
#2680=EDGE_CURVE('',#2231,#2232,#1308,.T.);
#2681=EDGE_CURVE('',#2233,#2234,#1309,.T.);
#2682=EDGE_CURVE('',#2235,#2233,#1310,.T.);
#2683=EDGE_CURVE('',#2234,#2235,#1311,.T.);
#2684=EDGE_CURVE('',#2234,#2236,#1376,.T.);
#2685=EDGE_CURVE('',#2237,#2236,#1312,.T.);
#2686=EDGE_CURVE('',#2238,#2237,#1313,.T.);
#2687=EDGE_CURVE('',#2236,#2238,#1314,.T.);
#2688=EDGE_CURVE('',#2239,#2240,#1315,.T.);
#2689=EDGE_CURVE('',#2240,#2239,#1316,.T.);
#2690=EDGE_CURVE('',#2240,#2241,#1377,.T.);
#2691=EDGE_CURVE('',#2242,#2241,#1317,.T.);
#2692=EDGE_CURVE('',#2241,#2242,#1318,.T.);
#2693=EDGE_CURVE('',#2243,#2243,#1947,.T.);
#2694=EDGE_CURVE('',#2243,#2217,#1378,.T.);
#2695=EDGE_CURVE('',#2216,#2227,#1379,.T.);
#2696=EDGE_CURVE('',#2226,#2237,#1380,.T.);
#2697=EDGE_CURVE('',#2236,#2244,#1381,.T.);
#2698=EDGE_CURVE('',#2244,#2244,#1948,.T.);
#2699=EDGE_CURVE('',#2245,#2245,#1949,.T.);
#2700=EDGE_CURVE('',#2245,#2246,#1382,.T.);
#2701=EDGE_CURVE('',#2246,#2246,#1950,.T.);
#2702=EDGE_CURVE('',#2247,#2247,#1951,.T.);
#2703=EDGE_CURVE('',#2247,#2234,#1383,.T.);
#2704=EDGE_CURVE('',#2235,#2224,#1384,.T.);
#2705=EDGE_CURVE('',#2225,#2214,#1385,.T.);
#2706=EDGE_CURVE('',#2215,#2248,#1386,.T.);
#2707=EDGE_CURVE('',#2248,#2248,#1952,.T.);
#3367=ORIENTED_EDGE('',*,*,#2639,.F.);
#3368=ORIENTED_EDGE('',*,*,#2640,.T.);
#3369=ORIENTED_EDGE('',*,*,#2641,.F.);
#3370=ORIENTED_EDGE('',*,*,#2640,.F.);
#3371=ORIENTED_EDGE('',*,*,#2642,.F.);
#3372=ORIENTED_EDGE('',*,*,#2643,.T.);
#3373=ORIENTED_EDGE('',*,*,#2644,.F.);
#3374=ORIENTED_EDGE('',*,*,#2643,.F.);
#3375=ORIENTED_EDGE('',*,*,#2645,.F.);
#3376=ORIENTED_EDGE('',*,*,#2646,.T.);
#3377=ORIENTED_EDGE('',*,*,#2647,.F.);
#3378=ORIENTED_EDGE('',*,*,#2646,.F.);
#3379=ORIENTED_EDGE('',*,*,#2648,.F.);
#3380=ORIENTED_EDGE('',*,*,#2649,.T.);
#3381=ORIENTED_EDGE('',*,*,#2650,.F.);
#3382=ORIENTED_EDGE('',*,*,#2649,.F.);
#3383=ORIENTED_EDGE('',*,*,#2651,.F.);
#3384=ORIENTED_EDGE('',*,*,#2652,.T.);
#3385=ORIENTED_EDGE('',*,*,#2653,.F.);
#3386=ORIENTED_EDGE('',*,*,#2652,.F.);
#3387=ORIENTED_EDGE('',*,*,#2654,.F.);
#3388=ORIENTED_EDGE('',*,*,#2655,.T.);
#3389=ORIENTED_EDGE('',*,*,#2656,.F.);
#3390=ORIENTED_EDGE('',*,*,#2655,.F.);
#3391=ORIENTED_EDGE('',*,*,#2657,.F.);
#3392=ORIENTED_EDGE('',*,*,#2658,.F.);
#3393=ORIENTED_EDGE('',*,*,#2659,.F.);
#3394=ORIENTED_EDGE('',*,*,#2660,.T.);
#3395=ORIENTED_EDGE('',*,*,#2661,.F.);
#3396=ORIENTED_EDGE('',*,*,#2662,.F.);
#3397=ORIENTED_EDGE('',*,*,#2663,.F.);
#3398=ORIENTED_EDGE('',*,*,#2660,.F.);
#3399=ORIENTED_EDGE('',*,*,#2664,.F.);
#3400=ORIENTED_EDGE('',*,*,#2665,.F.);
#3401=ORIENTED_EDGE('',*,*,#2666,.T.);
#3402=ORIENTED_EDGE('',*,*,#2667,.F.);
#3403=ORIENTED_EDGE('',*,*,#2668,.F.);
#3404=ORIENTED_EDGE('',*,*,#2666,.F.);
#3405=ORIENTED_EDGE('',*,*,#2669,.F.);
#3406=ORIENTED_EDGE('',*,*,#2670,.F.);
#3407=ORIENTED_EDGE('',*,*,#2671,.F.);
#3408=ORIENTED_EDGE('',*,*,#2672,.T.);
#3409=ORIENTED_EDGE('',*,*,#2673,.F.);
#3410=ORIENTED_EDGE('',*,*,#2674,.F.);
#3411=ORIENTED_EDGE('',*,*,#2675,.F.);
#3412=ORIENTED_EDGE('',*,*,#2672,.F.);
#3413=ORIENTED_EDGE('',*,*,#2676,.F.);
#3414=ORIENTED_EDGE('',*,*,#2677,.F.);
#3415=ORIENTED_EDGE('',*,*,#2678,.T.);
#3416=ORIENTED_EDGE('',*,*,#2679,.F.);
#3417=ORIENTED_EDGE('',*,*,#2680,.F.);
#3418=ORIENTED_EDGE('',*,*,#2678,.F.);
#3419=ORIENTED_EDGE('',*,*,#2681,.F.);
#3420=ORIENTED_EDGE('',*,*,#2682,.F.);
#3421=ORIENTED_EDGE('',*,*,#2683,.F.);
#3422=ORIENTED_EDGE('',*,*,#2684,.T.);
#3423=ORIENTED_EDGE('',*,*,#2685,.F.);
#3424=ORIENTED_EDGE('',*,*,#2686,.F.);
#3425=ORIENTED_EDGE('',*,*,#2687,.F.);
#3426=ORIENTED_EDGE('',*,*,#2684,.F.);
#3427=ORIENTED_EDGE('',*,*,#2688,.F.);
#3428=ORIENTED_EDGE('',*,*,#2689,.F.);
#3429=ORIENTED_EDGE('',*,*,#2690,.T.);
#3430=ORIENTED_EDGE('',*,*,#2691,.F.);
#3431=ORIENTED_EDGE('',*,*,#2692,.F.);
#3432=ORIENTED_EDGE('',*,*,#2690,.F.);
#3433=ORIENTED_EDGE('',*,*,#2693,.F.);
#3434=ORIENTED_EDGE('',*,*,#2694,.T.);
#3435=ORIENTED_EDGE('',*,*,#2661,.T.);
#3436=ORIENTED_EDGE('',*,*,#2695,.T.);
#3437=ORIENTED_EDGE('',*,*,#2673,.T.);
#3438=ORIENTED_EDGE('',*,*,#2696,.T.);
#3439=ORIENTED_EDGE('',*,*,#2685,.T.);
#3440=ORIENTED_EDGE('',*,*,#2697,.T.);
#3441=ORIENTED_EDGE('',*,*,#2698,.F.);
#3442=ORIENTED_EDGE('',*,*,#2697,.F.);
#3443=ORIENTED_EDGE('',*,*,#2687,.T.);
#3444=ORIENTED_EDGE('',*,*,#2686,.T.);
#3445=ORIENTED_EDGE('',*,*,#2696,.F.);
#3446=ORIENTED_EDGE('',*,*,#2675,.T.);
#3447=ORIENTED_EDGE('',*,*,#2674,.T.);
#3448=ORIENTED_EDGE('',*,*,#2695,.F.);
#3449=ORIENTED_EDGE('',*,*,#2663,.T.);
#3450=ORIENTED_EDGE('',*,*,#2662,.T.);
#3451=ORIENTED_EDGE('',*,*,#2694,.F.);
#3452=ORIENTED_EDGE('',*,*,#2642,.T.);
#3453=ORIENTED_EDGE('',*,*,#2641,.T.);
#3454=ORIENTED_EDGE('',*,*,#2648,.T.);
#3455=ORIENTED_EDGE('',*,*,#2647,.T.);
#3456=ORIENTED_EDGE('',*,*,#2654,.T.);
#3457=ORIENTED_EDGE('',*,*,#2653,.T.);
#3458=ORIENTED_EDGE('',*,*,#2664,.T.);
#3459=ORIENTED_EDGE('',*,*,#2665,.T.);
#3460=ORIENTED_EDGE('',*,*,#2676,.T.);
#3461=ORIENTED_EDGE('',*,*,#2677,.T.);
#3462=ORIENTED_EDGE('',*,*,#2688,.T.);
#3463=ORIENTED_EDGE('',*,*,#2689,.T.);
#3464=ORIENTED_EDGE('',*,*,#2693,.T.);
#3465=ORIENTED_EDGE('',*,*,#2699,.F.);
#3466=ORIENTED_EDGE('',*,*,#2700,.T.);
#3467=ORIENTED_EDGE('',*,*,#2701,.F.);
#3468=ORIENTED_EDGE('',*,*,#2700,.F.);
#3469=ORIENTED_EDGE('',*,*,#2699,.T.);
#3470=ORIENTED_EDGE('',*,*,#2698,.T.);
#3471=ORIENTED_EDGE('',*,*,#2702,.F.);
#3472=ORIENTED_EDGE('',*,*,#2703,.T.);
#3473=ORIENTED_EDGE('',*,*,#2683,.T.);
#3474=ORIENTED_EDGE('',*,*,#2704,.T.);
#3475=ORIENTED_EDGE('',*,*,#2671,.T.);
#3476=ORIENTED_EDGE('',*,*,#2705,.T.);
#3477=ORIENTED_EDGE('',*,*,#2659,.T.);
#3478=ORIENTED_EDGE('',*,*,#2706,.T.);
#3479=ORIENTED_EDGE('',*,*,#2707,.T.);
#3480=ORIENTED_EDGE('',*,*,#2706,.F.);
#3481=ORIENTED_EDGE('',*,*,#2658,.T.);
#3482=ORIENTED_EDGE('',*,*,#2657,.T.);
#3483=ORIENTED_EDGE('',*,*,#2705,.F.);
#3484=ORIENTED_EDGE('',*,*,#2670,.T.);
#3485=ORIENTED_EDGE('',*,*,#2669,.T.);
#3486=ORIENTED_EDGE('',*,*,#2704,.F.);
#3487=ORIENTED_EDGE('',*,*,#2682,.T.);
#3488=ORIENTED_EDGE('',*,*,#2681,.T.);
#3489=ORIENTED_EDGE('',*,*,#2703,.F.);
#3490=ORIENTED_EDGE('',*,*,#2644,.T.);
#3491=ORIENTED_EDGE('',*,*,#2639,.T.);
#3492=ORIENTED_EDGE('',*,*,#2650,.T.);
#3493=ORIENTED_EDGE('',*,*,#2645,.T.);
#3494=ORIENTED_EDGE('',*,*,#2656,.T.);
#3495=ORIENTED_EDGE('',*,*,#2651,.T.);
#3496=ORIENTED_EDGE('',*,*,#2667,.T.);
#3497=ORIENTED_EDGE('',*,*,#2668,.T.);
#3498=ORIENTED_EDGE('',*,*,#2679,.T.);
#3499=ORIENTED_EDGE('',*,*,#2680,.T.);
#3500=ORIENTED_EDGE('',*,*,#2691,.T.);
#3501=ORIENTED_EDGE('',*,*,#2692,.T.);
#3502=ORIENTED_EDGE('',*,*,#2702,.T.);
#3503=ORIENTED_EDGE('',*,*,#2701,.T.);
#3504=ORIENTED_EDGE('',*,*,#2707,.F.);
#4326=CYLINDRICAL_SURFACE('',#5119,0.05);
#4327=CYLINDRICAL_SURFACE('',#5120,0.05);
#4328=CYLINDRICAL_SURFACE('',#5121,0.05);
#4329=CYLINDRICAL_SURFACE('',#5122,0.05);
#4330=CYLINDRICAL_SURFACE('',#5123,0.05);
#4331=CYLINDRICAL_SURFACE('',#5124,0.05);
#4332=CYLINDRICAL_SURFACE('',#5125,0.0499999999999998);
#4333=CYLINDRICAL_SURFACE('',#5126,0.0499999999999998);
#4334=CYLINDRICAL_SURFACE('',#5127,0.05);
#4335=CYLINDRICAL_SURFACE('',#5128,0.05);
#4336=CYLINDRICAL_SURFACE('',#5129,0.05);
#4337=CYLINDRICAL_SURFACE('',#5130,0.05);
#4338=CYLINDRICAL_SURFACE('',#5131,0.4);
#4339=CYLINDRICAL_SURFACE('',#5135,0.6185);
#4340=CYLINDRICAL_SURFACE('',#5139,1.2);
#4473=ADVANCED_FACE('',(#638),#4326,.F.);
#4474=ADVANCED_FACE('',(#639),#4327,.F.);
#4475=ADVANCED_FACE('',(#640),#4328,.F.);
#4476=ADVANCED_FACE('',(#641),#4329,.F.);
#4477=ADVANCED_FACE('',(#642),#4330,.F.);
#4478=ADVANCED_FACE('',(#643),#4331,.F.);
#4479=ADVANCED_FACE('',(#644),#4332,.F.);
#4480=ADVANCED_FACE('',(#645),#4333,.F.);
#4481=ADVANCED_FACE('',(#646),#4334,.F.);
#4482=ADVANCED_FACE('',(#647),#4335,.F.);
#4483=ADVANCED_FACE('',(#648),#4336,.F.);
#4484=ADVANCED_FACE('',(#649),#4337,.F.);
#4485=ADVANCED_FACE('',(#650,#325,#326,#327,#328,#329,#330,#331,#332,#333),
#4338,.F.);
#4486=ADVANCED_FACE('',(#651),#451,.T.);
#4487=ADVANCED_FACE('',(#652),#4339,.T.);
#4488=ADVANCED_FACE('',(#653,#334),#452,.T.);
#4489=ADVANCED_FACE('',(#654,#335,#336,#337,#338,#339,#340,#341,#342,#343),
#4340,.T.);
#4490=ADVANCED_FACE('',(#655,#344),#453,.T.);
#4491=ADVANCED_FACE('',(#656),#454,.F.);
#4691=CLOSED_SHELL('',(#4473,#4474,#4475,#4476,#4477,#4478,#4479,#4480,
#4481,#4482,#4483,#4484,#4485,#4486,#4487,#4488,#4489,#4490,#4491));
#5118=AXIS2_PLACEMENT_3D('',#7514,#5895,#5896);
#5119=AXIS2_PLACEMENT_3D('',#7515,#5897,#5898);
#5120=AXIS2_PLACEMENT_3D('',#7587,#5900,#5901);
#5121=AXIS2_PLACEMENT_3D('',#7659,#5903,#5904);
#5122=AXIS2_PLACEMENT_3D('',#7731,#5906,#5907);
#5123=AXIS2_PLACEMENT_3D('',#7803,#5909,#5910);
#5124=AXIS2_PLACEMENT_3D('',#7875,#5912,#5913);
#5125=AXIS2_PLACEMENT_3D('',#7947,#5915,#5916);
#5126=AXIS2_PLACEMENT_3D('',#8031,#5918,#5919);
#5127=AXIS2_PLACEMENT_3D('',#8109,#5921,#5922);
#5128=AXIS2_PLACEMENT_3D('',#8193,#5924,#5925);
#5129=AXIS2_PLACEMENT_3D('',#8271,#5927,#5928);
#5130=AXIS2_PLACEMENT_3D('',#8355,#5930,#5931);
#5131=AXIS2_PLACEMENT_3D('',#8433,#5933,#5934);
#5132=AXIS2_PLACEMENT_3D('',#8435,#5935,#5936);
#5133=AXIS2_PLACEMENT_3D('',#8441,#5941,#5942);
#5134=AXIS2_PLACEMENT_3D('',#8442,#5943,#5944);
#5135=AXIS2_PLACEMENT_3D('',#8443,#5945,#5946);
#5136=AXIS2_PLACEMENT_3D('',#8445,#5947,#5948);
#5137=AXIS2_PLACEMENT_3D('',#8448,#5950,#5951);
#5138=AXIS2_PLACEMENT_3D('',#8449,#5952,#5953);
#5139=AXIS2_PLACEMENT_3D('',#8450,#5954,#5955);
#5140=AXIS2_PLACEMENT_3D('',#8452,#5956,#5957);
#5141=AXIS2_PLACEMENT_3D('',#8458,#5962,#5963);
#5142=AXIS2_PLACEMENT_3D('',#8459,#5964,#5965);
#5143=AXIS2_PLACEMENT_3D('',#8460,#5966,#5967);
#5895=DIRECTION('axis',(0.,0.,1.));
#5896=DIRECTION('refdir',(1.,0.,0.));
#5897=DIRECTION('center_axis',(0.,1.,0.));
#5898=DIRECTION('ref_axis',(1.,0.,0.));
#5899=DIRECTION('',(0.,1.,0.));
#5900=DIRECTION('center_axis',(0.,1.,0.));
#5901=DIRECTION('ref_axis',(1.,0.,0.));
#5902=DIRECTION('',(0.,1.,0.));
#5903=DIRECTION('center_axis',(0.,1.,0.));
#5904=DIRECTION('ref_axis',(1.,0.,0.));
#5905=DIRECTION('',(0.,1.,0.));
#5906=DIRECTION('center_axis',(0.,1.,0.));
#5907=DIRECTION('ref_axis',(1.,0.,0.));
#5908=DIRECTION('',(0.,1.,0.));
#5909=DIRECTION('center_axis',(0.,1.,0.));
#5910=DIRECTION('ref_axis',(1.,0.,0.));
#5911=DIRECTION('',(0.,1.,0.));
#5912=DIRECTION('center_axis',(0.,1.,0.));
#5913=DIRECTION('ref_axis',(1.,0.,0.));
#5914=DIRECTION('',(0.,1.,0.));
#5915=DIRECTION('center_axis',(1.,0.,0.));
#5916=DIRECTION('ref_axis',(0.,0.,-1.));
#5917=DIRECTION('',(1.,0.,0.));
#5918=DIRECTION('center_axis',(1.,0.,0.));
#5919=DIRECTION('ref_axis',(0.,0.,-1.));
#5920=DIRECTION('',(1.,0.,0.));
#5921=DIRECTION('center_axis',(1.,0.,0.));
#5922=DIRECTION('ref_axis',(0.,0.,-1.));
#5923=DIRECTION('',(1.,0.,0.));
#5924=DIRECTION('center_axis',(1.,0.,0.));
#5925=DIRECTION('ref_axis',(0.,0.,-1.));
#5926=DIRECTION('',(1.,0.,0.));
#5927=DIRECTION('center_axis',(1.,0.,0.));
#5928=DIRECTION('ref_axis',(0.,0.,-1.));
#5929=DIRECTION('',(1.,0.,0.));
#5930=DIRECTION('center_axis',(1.,0.,0.));
#5931=DIRECTION('ref_axis',(0.,0.,-1.));
#5932=DIRECTION('',(1.,0.,0.));
#5933=DIRECTION('center_axis',(0.,0.,1.));
#5934=DIRECTION('ref_axis',(1.,0.,0.));
#5935=DIRECTION('center_axis',(0.,0.,1.));
#5936=DIRECTION('ref_axis',(1.,0.,0.));
#5937=DIRECTION('',(0.,0.,1.));
#5938=DIRECTION('',(0.,0.,1.));
#5939=DIRECTION('',(0.,0.,1.));
#5940=DIRECTION('',(0.,0.,1.));
#5941=DIRECTION('center_axis',(0.,0.,-1.));
#5942=DIRECTION('ref_axis',(1.,0.,0.));
#5943=DIRECTION('center_axis',(0.,0.,1.));
#5944=DIRECTION('ref_axis',(1.,0.,0.));
#5945=DIRECTION('center_axis',(0.,0.,1.));
#5946=DIRECTION('ref_axis',(1.,0.,0.));
#5947=DIRECTION('center_axis',(0.,0.,1.));
#5948=DIRECTION('ref_axis',(1.,0.,0.));
#5949=DIRECTION('',(0.,0.,-1.));
#5950=DIRECTION('center_axis',(0.,0.,-1.));
#5951=DIRECTION('ref_axis',(1.,0.,0.));
#5952=DIRECTION('center_axis',(0.,0.,1.));
#5953=DIRECTION('ref_axis',(1.,0.,0.));
#5954=DIRECTION('center_axis',(0.,0.,1.));
#5955=DIRECTION('ref_axis',(1.,0.,0.));
#5956=DIRECTION('center_axis',(0.,0.,1.));
#5957=DIRECTION('ref_axis',(1.,0.,0.));
#5958=DIRECTION('',(0.,0.,-1.));
#5959=DIRECTION('',(0.,0.,-1.));
#5960=DIRECTION('',(0.,0.,-1.));
#5961=DIRECTION('',(0.,0.,-1.));
#5962=DIRECTION('center_axis',(0.,0.,1.));
#5963=DIRECTION('ref_axis',(1.,0.,0.));
#5964=DIRECTION('center_axis',(0.,0.,1.));
#5965=DIRECTION('ref_axis',(1.,0.,0.));
#5966=DIRECTION('center_axis',(0.,0.,1.));
#5967=DIRECTION('ref_axis',(1.,0.,0.));
#7514=CARTESIAN_POINT('',(0.,0.,0.));
#7515=CARTESIAN_POINT('Origin',(0.,-1.3,-2.5));
#7516=CARTESIAN_POINT('',(-0.05,-1.19895788082818,-2.5));
#7517=CARTESIAN_POINT('Ctrl Pts',(-0.05,-1.19895788082818,-2.5));
#7518=CARTESIAN_POINT('Ctrl Pts',(-0.05,-1.19895788082818,-2.49372110852169));
#7519=CARTESIAN_POINT('Ctrl Pts',(-0.0487450133099081,-1.19901227819454,
-2.48702419537593));
#7520=CARTESIAN_POINT('Ctrl Pts',(-0.0436421041657014,-1.19920885850753,
-2.47470544370928));
#7521=CARTESIAN_POINT('Ctrl Pts',(-0.0397942217705328,-1.1993482149535,
-2.46908354365188));
#7522=CARTESIAN_POINT('Ctrl Pts',(-0.0309164568000038,-1.19960989221221,
-2.46020577868135));
#7523=CARTESIAN_POINT('Ctrl Pts',(-0.0252945565319674,-1.19974919586288,
-2.45635789595805));
#7524=CARTESIAN_POINT('Ctrl Pts',(-0.0129758042228731,-1.19994565546462,
-2.45125498650009));
#7525=CARTESIAN_POINT('Ctrl Pts',(-0.00627889083911039,-1.2,-2.45));
#7526=CARTESIAN_POINT('Ctrl Pts',(0.00627889083911038,-1.2,-2.45));
#7527=CARTESIAN_POINT('Ctrl Pts',(0.012975804222873,-1.19994565546462,-2.45125498650009));
#7528=CARTESIAN_POINT('Ctrl Pts',(0.0252945565319674,-1.19974919586288,
-2.45635789595805));
#7529=CARTESIAN_POINT('Ctrl Pts',(0.0309164568000038,-1.19960989221221,
-2.46020577868135));
#7530=CARTESIAN_POINT('Ctrl Pts',(0.0397942217705328,-1.1993482149535,-2.46908354365188));
#7531=CARTESIAN_POINT('Ctrl Pts',(0.0436421041657014,-1.19920885850753,
-2.47470544370928));
#7532=CARTESIAN_POINT('Ctrl Pts',(0.0487450133099081,-1.19901227819454,
-2.48702419537593));
#7533=CARTESIAN_POINT('Ctrl Pts',(0.05,-1.19895788082818,-2.49372110852169));
#7534=CARTESIAN_POINT('Ctrl Pts',(0.05,-1.19895788082818,-2.50627889147831));
#7535=CARTESIAN_POINT('Ctrl Pts',(0.0487450133099081,-1.19901227819454,
-2.51297580462407));
#7536=CARTESIAN_POINT('Ctrl Pts',(0.0436421041657014,-1.19920885850753,
-2.52529455629072));
#7537=CARTESIAN_POINT('Ctrl Pts',(0.0397942217705328,-1.1993482149535,-2.53091645634812));
#7538=CARTESIAN_POINT('Ctrl Pts',(0.0309164568000038,-1.19960989221221,
-2.53979422131865));
#7539=CARTESIAN_POINT('Ctrl Pts',(0.0252945565319675,-1.19974919586288,
-2.54364210404195));
#7540=CARTESIAN_POINT('Ctrl Pts',(0.0129758042228731,-1.19994565546462,
-2.54874501349991));
#7541=CARTESIAN_POINT('Ctrl Pts',(0.0062788908391104,-1.2,-2.55));
#7542=CARTESIAN_POINT('Ctrl Pts',(-0.00627889083911037,-1.2,-2.55));
#7543=CARTESIAN_POINT('Ctrl Pts',(-0.012975804222873,-1.19994565546462,
-2.54874501349991));
#7544=CARTESIAN_POINT('Ctrl Pts',(-0.0252945565319674,-1.19974919586288,
-2.54364210404195));
#7545=CARTESIAN_POINT('Ctrl Pts',(-0.0309164568000038,-1.19960989221221,
-2.53979422131865));
#7546=CARTESIAN_POINT('Ctrl Pts',(-0.0397942217705328,-1.1993482149535,
-2.53091645634812));
#7547=CARTESIAN_POINT('Ctrl Pts',(-0.0436421041657014,-1.19920885850753,
-2.52529455629072));
#7548=CARTESIAN_POINT('Ctrl Pts',(-0.0487450133099081,-1.19901227819454,
-2.51297580462407));
#7549=CARTESIAN_POINT('Ctrl Pts',(-0.05,-1.19895788082818,-2.50627889147831));
#7550=CARTESIAN_POINT('Ctrl Pts',(-0.05,-1.19895788082818,-2.5));
#7551=CARTESIAN_POINT('',(-0.05,-0.396862696659689,-2.5));
#7552=CARTESIAN_POINT('',(-0.05,-1.3,-2.5));
#7553=CARTESIAN_POINT('Ctrl Pts',(-0.05,-0.396862696659689,-2.5));
#7554=CARTESIAN_POINT('Ctrl Pts',(-0.05,-0.396862696659689,-2.50628520096426));
#7555=CARTESIAN_POINT('Ctrl Pts',(-0.0487425534891116,-0.397027412247524,
-2.51298480122901));
#7556=CARTESIAN_POINT('Ctrl Pts',(-0.0436378373878618,-0.397620851691571,
-2.52530179409386));
#7557=CARTESIAN_POINT('Ctrl Pts',(-0.0397909243921696,-0.398040841710914,
-2.53091975372649));
#7558=CARTESIAN_POINT('Ctrl Pts',(-0.0309197907817458,-0.398828027526425,
-2.53979088733691));
#7559=CARTESIAN_POINT('Ctrl Pts',(-0.0253018150396577,-0.399246581249293,
-2.5436378293633));
#7560=CARTESIAN_POINT('Ctrl Pts',(-0.0129847676279313,-0.399836729543542,
-2.5487425667586));
#7561=CARTESIAN_POINT('Ctrl Pts',(-0.00628514845714647,-0.4,-2.55));
#7562=CARTESIAN_POINT('Ctrl Pts',(0.00628514845714648,-0.4,-2.55));
#7563=CARTESIAN_POINT('Ctrl Pts',(0.012984767627931,-0.399836729543542,
-2.5487425667586));
#7564=CARTESIAN_POINT('Ctrl Pts',(0.0253018150396574,-0.399246581249293,
-2.5436378293633));
#7565=CARTESIAN_POINT('Ctrl Pts',(0.0309197907817458,-0.398828027526425,
-2.53979088733691));
#7566=CARTESIAN_POINT('Ctrl Pts',(0.0397909243921696,-0.398040841710914,
-2.53091975372649));
#7567=CARTESIAN_POINT('Ctrl Pts',(0.0436378373878616,-0.397620851691571,
-2.52530179409386));
#7568=CARTESIAN_POINT('Ctrl Pts',(0.0487425534891115,-0.397027412247524,
-2.51298480122901));
#7569=CARTESIAN_POINT('Ctrl Pts',(0.05,-0.396862696659689,-2.50628520096426));
#7570=CARTESIAN_POINT('Ctrl Pts',(0.05,-0.396862696659689,-2.49371479903574));
#7571=CARTESIAN_POINT('Ctrl Pts',(0.0487425534891116,-0.397027412247524,
-2.48701519877099));
#7572=CARTESIAN_POINT('Ctrl Pts',(0.0436378373878618,-0.397620851691571,
-2.47469820590614));
#7573=CARTESIAN_POINT('Ctrl Pts',(0.0397909243921696,-0.398040841710914,
-2.46908024627351));
#7574=CARTESIAN_POINT('Ctrl Pts',(0.0309197907817458,-0.398828027526425,
-2.46020911266309));
#7575=CARTESIAN_POINT('Ctrl Pts',(0.0253018150396577,-0.399246581249293,
-2.4563621706367));
#7576=CARTESIAN_POINT('Ctrl Pts',(0.0129847676279313,-0.399836729543542,
-2.4512574332414));
#7577=CARTESIAN_POINT('Ctrl Pts',(0.00628514845714648,-0.4,-2.45));
#7578=CARTESIAN_POINT('Ctrl Pts',(-0.00628514845714647,-0.4,-2.45));
#7579=CARTESIAN_POINT('Ctrl Pts',(-0.0129847676279313,-0.399836729543542,
-2.4512574332414));
#7580=CARTESIAN_POINT('Ctrl Pts',(-0.0253018150396577,-0.399246581249293,
-2.4563621706367));
#7581=CARTESIAN_POINT('Ctrl Pts',(-0.0309197907817458,-0.398828027526425,
-2.46020911266309));
#7582=CARTESIAN_POINT('Ctrl Pts',(-0.0397909243921696,-0.398040841710914,
-2.46908024627351));
#7583=CARTESIAN_POINT('Ctrl Pts',(-0.0436378373878618,-0.397620851691571,
-2.47469820590614));
#7584=CARTESIAN_POINT('Ctrl Pts',(-0.0487425534891116,-0.397027412247524,
-2.48701519877099));
#7585=CARTESIAN_POINT('Ctrl Pts',(-0.05,-0.396862696659689,-2.49371479903574));
#7586=CARTESIAN_POINT('Ctrl Pts',(-0.05,-0.396862696659689,-2.5));
#7587=CARTESIAN_POINT('Origin',(0.,-1.3,-2.5));
#7588=CARTESIAN_POINT('',(-0.05,0.396862696659689,-2.5));
#7589=CARTESIAN_POINT('Ctrl Pts',(-0.05,0.396862696659689,-2.5));
#7590=CARTESIAN_POINT('Ctrl Pts',(-0.05,0.396862696659689,-2.49371479903574));
#7591=CARTESIAN_POINT('Ctrl Pts',(-0.0487425534891116,0.397027412247524,
-2.48701519877099));
#7592=CARTESIAN_POINT('Ctrl Pts',(-0.0436378373878618,0.397620851691571,
-2.47469820590614));
#7593=CARTESIAN_POINT('Ctrl Pts',(-0.0397909243921696,0.398040841710914,
-2.46908024627351));
#7594=CARTESIAN_POINT('Ctrl Pts',(-0.0309197907817458,0.398828027526425,
-2.46020911266309));
#7595=CARTESIAN_POINT('Ctrl Pts',(-0.0253018150396577,0.399246581249293,
-2.4563621706367));
#7596=CARTESIAN_POINT('Ctrl Pts',(-0.0129847676279313,0.399836729543542,
-2.4512574332414));
#7597=CARTESIAN_POINT('Ctrl Pts',(-0.00628514845714647,0.4,-2.45));
#7598=CARTESIAN_POINT('Ctrl Pts',(0.00628514845714648,0.4,-2.45));
#7599=CARTESIAN_POINT('Ctrl Pts',(0.0129847676279313,0.399836729543542,
-2.4512574332414));
#7600=CARTESIAN_POINT('Ctrl Pts',(0.0253018150396577,0.399246581249293,
-2.4563621706367));
#7601=CARTESIAN_POINT('Ctrl Pts',(0.0309197907817458,0.398828027526425,
-2.46020911266309));
#7602=CARTESIAN_POINT('Ctrl Pts',(0.0397909243921696,0.398040841710914,
-2.46908024627351));
#7603=CARTESIAN_POINT('Ctrl Pts',(0.0436378373878621,0.397620851691571,
-2.47469820590614));
#7604=CARTESIAN_POINT('Ctrl Pts',(0.0487425534891117,0.397027412247524,
-2.48701519877099));
#7605=CARTESIAN_POINT('Ctrl Pts',(0.05,0.396862696659689,-2.49371479903574));
#7606=CARTESIAN_POINT('Ctrl Pts',(0.05,0.396862696659689,-2.50628520096426));
#7607=CARTESIAN_POINT('Ctrl Pts',(0.0487425534891116,0.397027412247524,
-2.51298480122901));
#7608=CARTESIAN_POINT('Ctrl Pts',(0.0436378373878618,0.397620851691571,
-2.52530179409386));
#7609=CARTESIAN_POINT('Ctrl Pts',(0.0397909243921696,0.398040841710914,
-2.53091975372649));
#7610=CARTESIAN_POINT('Ctrl Pts',(0.0309197907817458,0.398828027526425,
-2.53979088733691));
#7611=CARTESIAN_POINT('Ctrl Pts',(0.0253018150396574,0.399246581249293,
-2.5436378293633));
#7612=CARTESIAN_POINT('Ctrl Pts',(0.012984767627931,0.399836729543542,-2.5487425667586));
#7613=CARTESIAN_POINT('Ctrl Pts',(0.00628514845714648,0.4,-2.55));
#7614=CARTESIAN_POINT('Ctrl Pts',(-0.00628514845714647,0.4,-2.55));
#7615=CARTESIAN_POINT('Ctrl Pts',(-0.012984767627931,0.399836729543542,
-2.5487425667586));
#7616=CARTESIAN_POINT('Ctrl Pts',(-0.0253018150396574,0.399246581249293,
-2.5436378293633));
#7617=CARTESIAN_POINT('Ctrl Pts',(-0.0309197907817458,0.398828027526425,
-2.53979088733691));
#7618=CARTESIAN_POINT('Ctrl Pts',(-0.0397909243921696,0.398040841710914,
-2.53091975372649));
#7619=CARTESIAN_POINT('Ctrl Pts',(-0.0436378373878618,0.397620851691571,
-2.52530179409386));
#7620=CARTESIAN_POINT('Ctrl Pts',(-0.0487425534891116,0.397027412247524,
-2.51298480122901));
#7621=CARTESIAN_POINT('Ctrl Pts',(-0.05,0.396862696659689,-2.50628520096426));
#7622=CARTESIAN_POINT('Ctrl Pts',(-0.05,0.396862696659689,-2.5));
#7623=CARTESIAN_POINT('',(-0.05,1.19895788082818,-2.5));
#7624=CARTESIAN_POINT('',(-0.05,-1.3,-2.5));
#7625=CARTESIAN_POINT('Ctrl Pts',(-0.05,1.19895788082818,-2.5));
#7626=CARTESIAN_POINT('Ctrl Pts',(-0.05,1.19895788082818,-2.50627889147831));
#7627=CARTESIAN_POINT('Ctrl Pts',(-0.0487450133099081,1.19901227819454,
-2.51297580462407));
#7628=CARTESIAN_POINT('Ctrl Pts',(-0.0436421041657014,1.19920885850753,
-2.52529455629072));
#7629=CARTESIAN_POINT('Ctrl Pts',(-0.0397942217705328,1.1993482149535,-2.53091645634812));
#7630=CARTESIAN_POINT('Ctrl Pts',(-0.0309164568000038,1.19960989221221,
-2.53979422131865));
#7631=CARTESIAN_POINT('Ctrl Pts',(-0.0252945565319674,1.19974919586288,
-2.54364210404195));
#7632=CARTESIAN_POINT('Ctrl Pts',(-0.012975804222873,1.19994565546462,-2.54874501349991));
#7633=CARTESIAN_POINT('Ctrl Pts',(-0.00627889083911037,1.2,-2.55));
#7634=CARTESIAN_POINT('Ctrl Pts',(0.0062788908391104,1.2,-2.55));
#7635=CARTESIAN_POINT('Ctrl Pts',(0.0129758042228731,1.19994565546462,-2.54874501349991));
#7636=CARTESIAN_POINT('Ctrl Pts',(0.0252945565319675,1.19974919586288,-2.54364210404195));
#7637=CARTESIAN_POINT('Ctrl Pts',(0.0309164568000038,1.19960989221221,-2.53979422131865));
#7638=CARTESIAN_POINT('Ctrl Pts',(0.0397942217705328,1.1993482149535,-2.53091645634812));
#7639=CARTESIAN_POINT('Ctrl Pts',(0.0436421041657014,1.19920885850753,-2.52529455629072));
#7640=CARTESIAN_POINT('Ctrl Pts',(0.0487450133099081,1.19901227819454,-2.51297580462407));
#7641=CARTESIAN_POINT('Ctrl Pts',(0.05,1.19895788082818,-2.50627889147831));
#7642=CARTESIAN_POINT('Ctrl Pts',(0.05,1.19895788082818,-2.49372110852169));
#7643=CARTESIAN_POINT('Ctrl Pts',(0.0487450133099081,1.19901227819454,-2.48702419537593));
#7644=CARTESIAN_POINT('Ctrl Pts',(0.0436421041657014,1.19920885850753,-2.47470544370928));
#7645=CARTESIAN_POINT('Ctrl Pts',(0.0397942217705328,1.1993482149535,-2.46908354365188));
#7646=CARTESIAN_POINT('Ctrl Pts',(0.0309164568000038,1.19960989221221,-2.46020577868135));
#7647=CARTESIAN_POINT('Ctrl Pts',(0.0252945565319674,1.19974919586288,-2.45635789595805));
#7648=CARTESIAN_POINT('Ctrl Pts',(0.012975804222873,1.19994565546462,-2.45125498650009));
#7649=CARTESIAN_POINT('Ctrl Pts',(0.00627889083911038,1.2,-2.45));
#7650=CARTESIAN_POINT('Ctrl Pts',(-0.00627889083911039,1.2,-2.45));
#7651=CARTESIAN_POINT('Ctrl Pts',(-0.0129758042228731,1.19994565546462,
-2.45125498650009));
#7652=CARTESIAN_POINT('Ctrl Pts',(-0.0252945565319674,1.19974919586288,
-2.45635789595805));
#7653=CARTESIAN_POINT('Ctrl Pts',(-0.0309164568000038,1.19960989221221,
-2.46020577868135));
#7654=CARTESIAN_POINT('Ctrl Pts',(-0.0397942217705328,1.1993482149535,-2.46908354365188));
#7655=CARTESIAN_POINT('Ctrl Pts',(-0.0436421041657014,1.19920885850753,
-2.47470544370928));
#7656=CARTESIAN_POINT('Ctrl Pts',(-0.0487450133099081,1.19901227819454,
-2.48702419537593));
#7657=CARTESIAN_POINT('Ctrl Pts',(-0.05,1.19895788082818,-2.49372110852169));
#7658=CARTESIAN_POINT('Ctrl Pts',(-0.05,1.19895788082818,-2.5));
#7659=CARTESIAN_POINT('Origin',(0.,-1.3,-1.5));
#7660=CARTESIAN_POINT('',(-0.05,-1.19895788082818,-1.5));
#7661=CARTESIAN_POINT('Ctrl Pts',(-0.05,-1.19895788082818,-1.5));
#7662=CARTESIAN_POINT('Ctrl Pts',(-0.05,-1.19895788082818,-1.49372110852169));
#7663=CARTESIAN_POINT('Ctrl Pts',(-0.0487450133099081,-1.19901227819454,
-1.48702419537594));
#7664=CARTESIAN_POINT('Ctrl Pts',(-0.0436421041657014,-1.19920885850753,
-1.47470544370928));
#7665=CARTESIAN_POINT('Ctrl Pts',(-0.0397942217705328,-1.1993482149535,
-1.46908354365188));
#7666=CARTESIAN_POINT('Ctrl Pts',(-0.0309164568000038,-1.19960989221221,
-1.46020577868135));
#7667=CARTESIAN_POINT('Ctrl Pts',(-0.0252945565319674,-1.19974919586288,
-1.45635789595805));
#7668=CARTESIAN_POINT('Ctrl Pts',(-0.012975804222873,-1.19994565546462,
-1.45125498650009));
#7669=CARTESIAN_POINT('Ctrl Pts',(-0.00627889083911039,-1.2,-1.45));
#7670=CARTESIAN_POINT('Ctrl Pts',(0.00627889083911038,-1.2,-1.45));
#7671=CARTESIAN_POINT('Ctrl Pts',(0.012975804222873,-1.19994565546462,-1.45125498650009));
#7672=CARTESIAN_POINT('Ctrl Pts',(0.0252945565319674,-1.19974919586288,
-1.45635789595805));
#7673=CARTESIAN_POINT('Ctrl Pts',(0.0309164568000038,-1.19960989221221,
-1.46020577868135));
#7674=CARTESIAN_POINT('Ctrl Pts',(0.0397942217705328,-1.1993482149535,-1.46908354365188));
#7675=CARTESIAN_POINT('Ctrl Pts',(0.0436421041657014,-1.19920885850753,
-1.47470544370928));
#7676=CARTESIAN_POINT('Ctrl Pts',(0.0487450133099081,-1.19901227819454,
-1.48702419537594));
#7677=CARTESIAN_POINT('Ctrl Pts',(0.05,-1.19895788082818,-1.49372110852169));
#7678=CARTESIAN_POINT('Ctrl Pts',(0.05,-1.19895788082818,-1.50627889147831));
#7679=CARTESIAN_POINT('Ctrl Pts',(0.0487450133099081,-1.19901227819454,
-1.51297580462406));
#7680=CARTESIAN_POINT('Ctrl Pts',(0.0436421041657014,-1.19920885850753,
-1.52529455629072));
#7681=CARTESIAN_POINT('Ctrl Pts',(0.0397942217705328,-1.1993482149535,-1.53091645634812));
#7682=CARTESIAN_POINT('Ctrl Pts',(0.0309164568000038,-1.19960989221221,
-1.53979422131865));
#7683=CARTESIAN_POINT('Ctrl Pts',(0.0252945565319674,-1.19974919586288,
-1.54364210404195));
#7684=CARTESIAN_POINT('Ctrl Pts',(0.0129758042228729,-1.19994565546462,
-1.54874501349991));
#7685=CARTESIAN_POINT('Ctrl Pts',(0.00627889083911041,-1.2,-1.55));
#7686=CARTESIAN_POINT('Ctrl Pts',(-0.00627889083911036,-1.2,-1.55));
#7687=CARTESIAN_POINT('Ctrl Pts',(-0.0129758042228728,-1.19994565546462,
-1.54874501349991));
#7688=CARTESIAN_POINT('Ctrl Pts',(-0.0252945565319673,-1.19974919586288,
-1.54364210404195));
#7689=CARTESIAN_POINT('Ctrl Pts',(-0.0309164568000037,-1.19960989221221,
-1.53979422131865));
#7690=CARTESIAN_POINT('Ctrl Pts',(-0.0397942217705328,-1.1993482149535,
-1.53091645634812));
#7691=CARTESIAN_POINT('Ctrl Pts',(-0.0436421041657014,-1.19920885850753,
-1.52529455629072));
#7692=CARTESIAN_POINT('Ctrl Pts',(-0.0487450133099081,-1.19901227819454,
-1.51297580462406));
#7693=CARTESIAN_POINT('Ctrl Pts',(-0.05,-1.19895788082818,-1.50627889147831));
#7694=CARTESIAN_POINT('Ctrl Pts',(-0.05,-1.19895788082818,-1.5));
#7695=CARTESIAN_POINT('',(-0.05,-0.396862696659689,-1.5));
#7696=CARTESIAN_POINT('',(-0.05,-1.3,-1.5));
#7697=CARTESIAN_POINT('Ctrl Pts',(-0.05,-0.396862696659689,-1.5));
#7698=CARTESIAN_POINT('Ctrl Pts',(-0.05,-0.396862696659689,-1.50628520096425));
#7699=CARTESIAN_POINT('Ctrl Pts',(-0.0487425534891115,-0.397027412247524,
-1.51298480122901));
#7700=CARTESIAN_POINT('Ctrl Pts',(-0.0436378373878619,-0.397620851691571,
-1.52530179409386));
#7701=CARTESIAN_POINT('Ctrl Pts',(-0.0397909243921696,-0.398040841710914,
-1.53091975372649));
#7702=CARTESIAN_POINT('Ctrl Pts',(-0.0309197907817458,-0.398828027526425,
-1.53979088733691));
#7703=CARTESIAN_POINT('Ctrl Pts',(-0.0253018150396575,-0.399246581249293,
-1.5436378293633));
#7704=CARTESIAN_POINT('Ctrl Pts',(-0.0129847676279312,-0.399836729543542,
-1.54874256675859));
#7705=CARTESIAN_POINT('Ctrl Pts',(-0.00628514845714648,-0.4,-1.55));
#7706=CARTESIAN_POINT('Ctrl Pts',(0.00628514845714648,-0.4,-1.55));
#7707=CARTESIAN_POINT('Ctrl Pts',(0.012984767627931,-0.399836729543542,
-1.54874256675859));
#7708=CARTESIAN_POINT('Ctrl Pts',(0.0253018150396574,-0.399246581249293,
-1.5436378293633));
#7709=CARTESIAN_POINT('Ctrl Pts',(0.0309197907817458,-0.398828027526425,
-1.53979088733691));
#7710=CARTESIAN_POINT('Ctrl Pts',(0.0397909243921696,-0.398040841710914,
-1.53091975372649));
#7711=CARTESIAN_POINT('Ctrl Pts',(0.0436378373878617,-0.397620851691571,
-1.52530179409386));
#7712=CARTESIAN_POINT('Ctrl Pts',(0.0487425534891115,-0.397027412247524,
-1.51298480122901));
#7713=CARTESIAN_POINT('Ctrl Pts',(0.05,-0.396862696659689,-1.50628520096426));
#7714=CARTESIAN_POINT('Ctrl Pts',(0.05,-0.396862696659689,-1.49371479903575));
#7715=CARTESIAN_POINT('Ctrl Pts',(0.0487425534891115,-0.397027412247524,
-1.48701519877099));
#7716=CARTESIAN_POINT('Ctrl Pts',(0.0436378373878619,-0.397620851691571,
-1.47469820590614));
#7717=CARTESIAN_POINT('Ctrl Pts',(0.0397909243921696,-0.398040841710914,
-1.46908024627351));
#7718=CARTESIAN_POINT('Ctrl Pts',(0.0309197907817458,-0.398828027526425,
-1.46020911266309));
#7719=CARTESIAN_POINT('Ctrl Pts',(0.0253018150396577,-0.399246581249293,
-1.4563621706367));
#7720=CARTESIAN_POINT('Ctrl Pts',(0.0129847676279313,-0.399836729543542,
-1.45125743324141));
#7721=CARTESIAN_POINT('Ctrl Pts',(0.00628514845714648,-0.4,-1.45));
#7722=CARTESIAN_POINT('Ctrl Pts',(-0.00628514845714647,-0.4,-1.45));
#7723=CARTESIAN_POINT('Ctrl Pts',(-0.0129847676279313,-0.399836729543542,
-1.45125743324141));
#7724=CARTESIAN_POINT('Ctrl Pts',(-0.0253018150396577,-0.399246581249293,
-1.4563621706367));
#7725=CARTESIAN_POINT('Ctrl Pts',(-0.0309197907817458,-0.398828027526425,
-1.46020911266309));
#7726=CARTESIAN_POINT('Ctrl Pts',(-0.0397909243921696,-0.398040841710914,
-1.46908024627351));
#7727=CARTESIAN_POINT('Ctrl Pts',(-0.0436378373878619,-0.397620851691571,
-1.47469820590614));
#7728=CARTESIAN_POINT('Ctrl Pts',(-0.0487425534891115,-0.397027412247524,
-1.48701519877099));
#7729=CARTESIAN_POINT('Ctrl Pts',(-0.05,-0.396862696659689,-1.49371479903575));
#7730=CARTESIAN_POINT('Ctrl Pts',(-0.05,-0.396862696659689,-1.5));
#7731=CARTESIAN_POINT('Origin',(0.,-1.3,-1.5));
#7732=CARTESIAN_POINT('',(-0.05,0.396862696659689,-1.5));
#7733=CARTESIAN_POINT('Ctrl Pts',(-0.05,0.396862696659689,-1.5));
#7734=CARTESIAN_POINT('Ctrl Pts',(-0.05,0.396862696659689,-1.49371479903575));
#7735=CARTESIAN_POINT('Ctrl Pts',(-0.0487425534891115,0.397027412247524,
-1.48701519877099));
#7736=CARTESIAN_POINT('Ctrl Pts',(-0.0436378373878619,0.397620851691571,
-1.47469820590614));
#7737=CARTESIAN_POINT('Ctrl Pts',(-0.0397909243921696,0.398040841710914,
-1.46908024627351));
#7738=CARTESIAN_POINT('Ctrl Pts',(-0.0309197907817458,0.398828027526425,
-1.46020911266309));
#7739=CARTESIAN_POINT('Ctrl Pts',(-0.0253018150396577,0.399246581249293,
-1.4563621706367));
#7740=CARTESIAN_POINT('Ctrl Pts',(-0.0129847676279313,0.399836729543542,
-1.4512574332414));
#7741=CARTESIAN_POINT('Ctrl Pts',(-0.00628514845714647,0.4,-1.45));
#7742=CARTESIAN_POINT('Ctrl Pts',(0.00628514845714648,0.4,-1.45));
#7743=CARTESIAN_POINT('Ctrl Pts',(0.0129847676279313,0.399836729543542,
-1.45125743324141));
#7744=CARTESIAN_POINT('Ctrl Pts',(0.0253018150396577,0.399246581249293,
-1.4563621706367));
#7745=CARTESIAN_POINT('Ctrl Pts',(0.0309197907817458,0.398828027526425,
-1.46020911266309));
#7746=CARTESIAN_POINT('Ctrl Pts',(0.0397909243921696,0.398040841710914,
-1.46908024627351));
#7747=CARTESIAN_POINT('Ctrl Pts',(0.0436378373878621,0.397620851691571,
-1.47469820590614));
#7748=CARTESIAN_POINT('Ctrl Pts',(0.0487425534891116,0.397027412247524,
-1.48701519877099));
#7749=CARTESIAN_POINT('Ctrl Pts',(0.05,0.396862696659689,-1.49371479903575));
#7750=CARTESIAN_POINT('Ctrl Pts',(0.05,0.396862696659689,-1.50628520096425));
#7751=CARTESIAN_POINT('Ctrl Pts',(0.0487425534891115,0.397027412247524,
-1.51298480122901));
#7752=CARTESIAN_POINT('Ctrl Pts',(0.0436378373878619,0.397620851691571,
-1.52530179409386));
#7753=CARTESIAN_POINT('Ctrl Pts',(0.0397909243921696,0.398040841710914,
-1.53091975372649));
#7754=CARTESIAN_POINT('Ctrl Pts',(0.0309197907817458,0.398828027526425,
-1.53979088733691));
#7755=CARTESIAN_POINT('Ctrl Pts',(0.0253018150396575,0.399246581249293,
-1.5436378293633));
#7756=CARTESIAN_POINT('Ctrl Pts',(0.0129847676279312,0.399836729543542,
-1.54874256675859));
#7757=CARTESIAN_POINT('Ctrl Pts',(0.00628514845714648,0.4,-1.55));
#7758=CARTESIAN_POINT('Ctrl Pts',(-0.00628514845714648,0.4,-1.55));
#7759=CARTESIAN_POINT('Ctrl Pts',(-0.0129847676279312,0.399836729543542,
-1.54874256675859));
#7760=CARTESIAN_POINT('Ctrl Pts',(-0.0253018150396575,0.399246581249293,
-1.5436378293633));
#7761=CARTESIAN_POINT('Ctrl Pts',(-0.0309197907817458,0.398828027526425,
-1.53979088733691));
#7762=CARTESIAN_POINT('Ctrl Pts',(-0.0397909243921696,0.398040841710914,
-1.53091975372648));
#7763=CARTESIAN_POINT('Ctrl Pts',(-0.043637837387862,0.397620851691571,
-1.52530179409386));
#7764=CARTESIAN_POINT('Ctrl Pts',(-0.0487425534891116,0.397027412247524,
-1.51298480122901));
#7765=CARTESIAN_POINT('Ctrl Pts',(-0.05,0.396862696659689,-1.50628520096425));
#7766=CARTESIAN_POINT('Ctrl Pts',(-0.05,0.396862696659689,-1.5));
#7767=CARTESIAN_POINT('',(-0.05,1.19895788082818,-1.5));
#7768=CARTESIAN_POINT('',(-0.05,-1.3,-1.5));
#7769=CARTESIAN_POINT('Ctrl Pts',(-0.05,1.19895788082818,-1.5));
#7770=CARTESIAN_POINT('Ctrl Pts',(-0.05,1.19895788082818,-1.50627889147831));
#7771=CARTESIAN_POINT('Ctrl Pts',(-0.0487450133099081,1.19901227819454,
-1.51297580462407));
#7772=CARTESIAN_POINT('Ctrl Pts',(-0.0436421041657012,1.19920885850753,
-1.52529455629072));
#7773=CARTESIAN_POINT('Ctrl Pts',(-0.0397942217705328,1.1993482149535,-1.53091645634812));
#7774=CARTESIAN_POINT('Ctrl Pts',(-0.0309164568000037,1.19960989221221,
-1.53979422131865));
#7775=CARTESIAN_POINT('Ctrl Pts',(-0.0252945565319673,1.19974919586288,
-1.54364210404195));
#7776=CARTESIAN_POINT('Ctrl Pts',(-0.0129758042228728,1.19994565546462,
-1.54874501349991));
#7777=CARTESIAN_POINT('Ctrl Pts',(-0.00627889083911036,1.2,-1.55));
#7778=CARTESIAN_POINT('Ctrl Pts',(0.00627889083911041,1.2,-1.55));
#7779=CARTESIAN_POINT('Ctrl Pts',(0.0129758042228726,1.19994565546462,-1.54874501349991));
#7780=CARTESIAN_POINT('Ctrl Pts',(0.0252945565319671,1.19974919586288,-1.54364210404195));
#7781=CARTESIAN_POINT('Ctrl Pts',(0.0309164568000038,1.19960989221221,-1.53979422131865));
#7782=CARTESIAN_POINT('Ctrl Pts',(0.0397942217705328,1.1993482149535,-1.53091645634812));
#7783=CARTESIAN_POINT('Ctrl Pts',(0.0436421041657012,1.19920885850753,-1.52529455629072));
#7784=CARTESIAN_POINT('Ctrl Pts',(0.048745013309908,1.19901227819454,-1.51297580462407));
#7785=CARTESIAN_POINT('Ctrl Pts',(0.05,1.19895788082818,-1.50627889147831));
#7786=CARTESIAN_POINT('Ctrl Pts',(0.05,1.19895788082818,-1.49372110852169));
#7787=CARTESIAN_POINT('Ctrl Pts',(0.0487450133099081,1.19901227819454,-1.48702419537594));
#7788=CARTESIAN_POINT('Ctrl Pts',(0.0436421041657014,1.19920885850753,-1.47470544370928));
#7789=CARTESIAN_POINT('Ctrl Pts',(0.0397942217705328,1.1993482149535,-1.46908354365188));
#7790=CARTESIAN_POINT('Ctrl Pts',(0.0309164568000038,1.19960989221221,-1.46020577868135));
#7791=CARTESIAN_POINT('Ctrl Pts',(0.0252945565319674,1.19974919586288,-1.45635789595805));
#7792=CARTESIAN_POINT('Ctrl Pts',(0.012975804222873,1.19994565546462,-1.45125498650009));
#7793=CARTESIAN_POINT('Ctrl Pts',(0.00627889083911038,1.2,-1.45));
#7794=CARTESIAN_POINT('Ctrl Pts',(-0.00627889083911039,1.2,-1.45));
#7795=CARTESIAN_POINT('Ctrl Pts',(-0.012975804222873,1.19994565546462,-1.45125498650009));
#7796=CARTESIAN_POINT('Ctrl Pts',(-0.0252945565319674,1.19974919586288,
-1.45635789595805));
#7797=CARTESIAN_POINT('Ctrl Pts',(-0.0309164568000038,1.19960989221221,
-1.46020577868135));
#7798=CARTESIAN_POINT('Ctrl Pts',(-0.0397942217705328,1.1993482149535,-1.46908354365188));
#7799=CARTESIAN_POINT('Ctrl Pts',(-0.0436421041657014,1.19920885850753,
-1.47470544370928));
#7800=CARTESIAN_POINT('Ctrl Pts',(-0.0487450133099081,1.19901227819454,
-1.48702419537594));
#7801=CARTESIAN_POINT('Ctrl Pts',(-0.05,1.19895788082818,-1.49372110852169));
#7802=CARTESIAN_POINT('Ctrl Pts',(-0.05,1.19895788082818,-1.5));
#7803=CARTESIAN_POINT('Origin',(0.,-1.3,-0.5));
#7804=CARTESIAN_POINT('',(-0.05,-1.19895788082818,-0.5));
#7805=CARTESIAN_POINT('Ctrl Pts',(-0.05,-1.19895788082818,-0.5));
#7806=CARTESIAN_POINT('Ctrl Pts',(-0.05,-1.19895788082818,-0.493721108521693));
#7807=CARTESIAN_POINT('Ctrl Pts',(-0.0487450133099082,-1.19901227819454,
-0.487024195375935));
#7808=CARTESIAN_POINT('Ctrl Pts',(-0.0436421041657013,-1.19920885850753,
-0.47470544370928));
#7809=CARTESIAN_POINT('Ctrl Pts',(-0.0397942217705328,-1.1993482149535,
-0.469083543651878));
#7810=CARTESIAN_POINT('Ctrl Pts',(-0.0309164568000038,-1.19960989221221,
-0.460205778681349));
#7811=CARTESIAN_POINT('Ctrl Pts',(-0.0252945565319674,-1.19974919586288,
-0.456357895958046));
#7812=CARTESIAN_POINT('Ctrl Pts',(-0.012975804222873,-1.19994565546462,
-0.451254986500089));
#7813=CARTESIAN_POINT('Ctrl Pts',(-0.00627889083911039,-1.2,-0.45));
#7814=CARTESIAN_POINT('Ctrl Pts',(0.00627889083911038,-1.2,-0.45));
#7815=CARTESIAN_POINT('Ctrl Pts',(0.012975804222873,-1.19994565546462,-0.451254986500089));
#7816=CARTESIAN_POINT('Ctrl Pts',(0.0252945565319674,-1.19974919586288,
-0.456357895958046));
#7817=CARTESIAN_POINT('Ctrl Pts',(0.0309164568000038,-1.19960989221221,
-0.460205778681349));
#7818=CARTESIAN_POINT('Ctrl Pts',(0.0397942217705328,-1.1993482149535,-0.469083543651878));
#7819=CARTESIAN_POINT('Ctrl Pts',(0.0436421041657013,-1.19920885850753,
-0.47470544370928));
#7820=CARTESIAN_POINT('Ctrl Pts',(0.0487450133099082,-1.19901227819454,
-0.487024195375935));
#7821=CARTESIAN_POINT('Ctrl Pts',(0.05,-1.19895788082818,-0.493721108521693));
#7822=CARTESIAN_POINT('Ctrl Pts',(0.05,-1.19895788082818,-0.506278891478307));
#7823=CARTESIAN_POINT('Ctrl Pts',(0.0487450133099082,-1.19901227819454,
-0.512975804624065));
#7824=CARTESIAN_POINT('Ctrl Pts',(0.0436421041657015,-1.19920885850753,
-0.52529455629072));
#7825=CARTESIAN_POINT('Ctrl Pts',(0.0397942217705327,-1.1993482149535,-0.530916456348121));
#7826=CARTESIAN_POINT('Ctrl Pts',(0.0309164568000038,-1.19960989221221,
-0.539794221318651));
#7827=CARTESIAN_POINT('Ctrl Pts',(0.0252945565319676,-1.19974919586288,
-0.543642104041954));
#7828=CARTESIAN_POINT('Ctrl Pts',(0.0129758042228732,-1.19994565546462,
-0.548745013499911));
#7829=CARTESIAN_POINT('Ctrl Pts',(0.00627889083911044,-1.2,-0.55));
#7830=CARTESIAN_POINT('Ctrl Pts',(-0.00627889083911041,-1.2,-0.55));
#7831=CARTESIAN_POINT('Ctrl Pts',(-0.0129758042228731,-1.19994565546462,
-0.548745013499911));
#7832=CARTESIAN_POINT('Ctrl Pts',(-0.0252945565319676,-1.19974919586288,
-0.543642104041954));
#7833=CARTESIAN_POINT('Ctrl Pts',(-0.0309164568000038,-1.19960989221221,
-0.539794221318651));
#7834=CARTESIAN_POINT('Ctrl Pts',(-0.0397942217705327,-1.1993482149535,
-0.530916456348121));
#7835=CARTESIAN_POINT('Ctrl Pts',(-0.0436421041657015,-1.19920885850753,
-0.52529455629072));
#7836=CARTESIAN_POINT('Ctrl Pts',(-0.0487450133099082,-1.19901227819454,
-0.512975804624065));
#7837=CARTESIAN_POINT('Ctrl Pts',(-0.05,-1.19895788082818,-0.506278891478307));
#7838=CARTESIAN_POINT('Ctrl Pts',(-0.05,-1.19895788082818,-0.5));
#7839=CARTESIAN_POINT('',(-0.05,-0.396862696659689,-0.5));
#7840=CARTESIAN_POINT('',(-0.05,-1.3,-0.5));
#7841=CARTESIAN_POINT('Ctrl Pts',(-0.05,-0.396862696659689,-0.5));
#7842=CARTESIAN_POINT('Ctrl Pts',(-0.05,-0.396862696659689,-0.506285200964255));
#7843=CARTESIAN_POINT('Ctrl Pts',(-0.0487425534891115,-0.397027412247524,
-0.512984801229014));
#7844=CARTESIAN_POINT('Ctrl Pts',(-0.0436378373878618,-0.397620851691571,
-0.525301794093861));
#7845=CARTESIAN_POINT('Ctrl Pts',(-0.0397909243921696,-0.398040841710914,
-0.530919753726485));
#7846=CARTESIAN_POINT('Ctrl Pts',(-0.0309197907817458,-0.398828027526425,
-0.539790887336909));
#7847=CARTESIAN_POINT('Ctrl Pts',(-0.0253018150396576,-0.399246581249293,
-0.543637829363298));
#7848=CARTESIAN_POINT('Ctrl Pts',(-0.0129847676279313,-0.399836729543542,
-0.548742566758595));
#7849=CARTESIAN_POINT('Ctrl Pts',(-0.00628514845714647,-0.4,-0.55));
#7850=CARTESIAN_POINT('Ctrl Pts',(0.00628514845714648,-0.4,-0.55));
#7851=CARTESIAN_POINT('Ctrl Pts',(0.0129847676279313,-0.399836729543542,
-0.548742566758595));
#7852=CARTESIAN_POINT('Ctrl Pts',(0.0253018150396576,-0.399246581249293,
-0.543637829363298));
#7853=CARTESIAN_POINT('Ctrl Pts',(0.0309197907817458,-0.398828027526425,
-0.539790887336909));
#7854=CARTESIAN_POINT('Ctrl Pts',(0.0397909243921696,-0.398040841710914,
-0.530919753726485));
#7855=CARTESIAN_POINT('Ctrl Pts',(0.0436378373878618,-0.397620851691571,
-0.525301794093861));
#7856=CARTESIAN_POINT('Ctrl Pts',(0.0487425534891115,-0.397027412247524,
-0.512984801229014));
#7857=CARTESIAN_POINT('Ctrl Pts',(0.05,-0.396862696659689,-0.506285200964255));
#7858=CARTESIAN_POINT('Ctrl Pts',(0.05,-0.396862696659689,-0.493714799035745));
#7859=CARTESIAN_POINT('Ctrl Pts',(0.0487425534891115,-0.397027412247524,
-0.487015198770986));
#7860=CARTESIAN_POINT('Ctrl Pts',(0.0436378373878618,-0.397620851691571,
-0.474698205906139));
#7861=CARTESIAN_POINT('Ctrl Pts',(0.0397909243921696,-0.398040841710914,
-0.469080246273515));
#7862=CARTESIAN_POINT('Ctrl Pts',(0.0309197907817458,-0.398828027526425,
-0.460209112663091));
#7863=CARTESIAN_POINT('Ctrl Pts',(0.0253018150396576,-0.399246581249293,
-0.456362170636702));
#7864=CARTESIAN_POINT('Ctrl Pts',(0.0129847676279313,-0.399836729543542,
-0.451257433241405));
#7865=CARTESIAN_POINT('Ctrl Pts',(0.00628514845714648,-0.4,-0.45));
#7866=CARTESIAN_POINT('Ctrl Pts',(-0.00628514845714647,-0.4,-0.45));
#7867=CARTESIAN_POINT('Ctrl Pts',(-0.0129847676279313,-0.399836729543542,
-0.451257433241405));
#7868=CARTESIAN_POINT('Ctrl Pts',(-0.0253018150396577,-0.399246581249293,
-0.456362170636702));
#7869=CARTESIAN_POINT('Ctrl Pts',(-0.0309197907817458,-0.398828027526425,
-0.460209112663091));
#7870=CARTESIAN_POINT('Ctrl Pts',(-0.0397909243921696,-0.398040841710914,
-0.469080246273515));
#7871=CARTESIAN_POINT('Ctrl Pts',(-0.0436378373878618,-0.397620851691571,
-0.474698205906139));
#7872=CARTESIAN_POINT('Ctrl Pts',(-0.0487425534891115,-0.397027412247524,
-0.487015198770986));
#7873=CARTESIAN_POINT('Ctrl Pts',(-0.05,-0.396862696659689,-0.493714799035745));
#7874=CARTESIAN_POINT('Ctrl Pts',(-0.05,-0.396862696659689,-0.5));
#7875=CARTESIAN_POINT('Origin',(0.,-1.3,-0.5));
#7876=CARTESIAN_POINT('',(-0.05,0.396862696659689,-0.5));
#7877=CARTESIAN_POINT('Ctrl Pts',(-0.05,0.396862696659689,-0.5));
#7878=CARTESIAN_POINT('Ctrl Pts',(-0.05,0.396862696659689,-0.493714799035745));
#7879=CARTESIAN_POINT('Ctrl Pts',(-0.0487425534891115,0.397027412247524,
-0.487015198770986));
#7880=CARTESIAN_POINT('Ctrl Pts',(-0.0436378373878618,0.397620851691571,
-0.474698205906139));
#7881=CARTESIAN_POINT('Ctrl Pts',(-0.0397909243921696,0.398040841710914,
-0.469080246273515));
#7882=CARTESIAN_POINT('Ctrl Pts',(-0.0309197907817458,0.398828027526425,
-0.460209112663091));
#7883=CARTESIAN_POINT('Ctrl Pts',(-0.0253018150396576,0.399246581249293,
-0.456362170636702));
#7884=CARTESIAN_POINT('Ctrl Pts',(-0.0129847676279312,0.399836729543542,
-0.451257433241405));
#7885=CARTESIAN_POINT('Ctrl Pts',(-0.00628514845714647,0.4,-0.45));
#7886=CARTESIAN_POINT('Ctrl Pts',(0.00628514845714648,0.4,-0.45));
#7887=CARTESIAN_POINT('Ctrl Pts',(0.0129847676279313,0.399836729543542,
-0.451257433241405));
#7888=CARTESIAN_POINT('Ctrl Pts',(0.0253018150396576,0.399246581249293,
-0.456362170636702));
#7889=CARTESIAN_POINT('Ctrl Pts',(0.0309197907817458,0.398828027526425,
-0.460209112663091));
#7890=CARTESIAN_POINT('Ctrl Pts',(0.0397909243921696,0.398040841710914,
-0.469080246273515));
#7891=CARTESIAN_POINT('Ctrl Pts',(0.0436378373878619,0.397620851691571,
-0.474698205906139));
#7892=CARTESIAN_POINT('Ctrl Pts',(0.0487425534891115,0.397027412247524,
-0.487015198770986));
#7893=CARTESIAN_POINT('Ctrl Pts',(0.05,0.396862696659689,-0.493714799035745));
#7894=CARTESIAN_POINT('Ctrl Pts',(0.05,0.396862696659689,-0.506285200964255));
#7895=CARTESIAN_POINT('Ctrl Pts',(0.0487425534891115,0.397027412247524,
-0.512984801229014));
#7896=CARTESIAN_POINT('Ctrl Pts',(0.0436378373878618,0.397620851691571,
-0.525301794093861));
#7897=CARTESIAN_POINT('Ctrl Pts',(0.0397909243921696,0.398040841710914,
-0.530919753726485));
#7898=CARTESIAN_POINT('Ctrl Pts',(0.0309197907817458,0.398828027526425,
-0.539790887336909));
#7899=CARTESIAN_POINT('Ctrl Pts',(0.0253018150396576,0.399246581249293,
-0.543637829363298));
#7900=CARTESIAN_POINT('Ctrl Pts',(0.0129847676279313,0.399836729543542,
-0.548742566758595));
#7901=CARTESIAN_POINT('Ctrl Pts',(0.00628514845714648,0.4,-0.55));
#7902=CARTESIAN_POINT('Ctrl Pts',(-0.00628514845714647,0.4,-0.55));
#7903=CARTESIAN_POINT('Ctrl Pts',(-0.0129847676279313,0.399836729543542,
-0.548742566758595));
#7904=CARTESIAN_POINT('Ctrl Pts',(-0.0253018150396576,0.399246581249293,
-0.543637829363298));
#7905=CARTESIAN_POINT('Ctrl Pts',(-0.0309197907817458,0.398828027526425,
-0.539790887336909));
#7906=CARTESIAN_POINT('Ctrl Pts',(-0.0397909243921696,0.398040841710914,
-0.530919753726485));
#7907=CARTESIAN_POINT('Ctrl Pts',(-0.0436378373878618,0.397620851691571,
-0.525301794093861));
#7908=CARTESIAN_POINT('Ctrl Pts',(-0.0487425534891115,0.397027412247524,
-0.512984801229014));
#7909=CARTESIAN_POINT('Ctrl Pts',(-0.05,0.396862696659689,-0.506285200964255));
#7910=CARTESIAN_POINT('Ctrl Pts',(-0.05,0.396862696659689,-0.5));
#7911=CARTESIAN_POINT('',(-0.05,1.19895788082818,-0.5));
#7912=CARTESIAN_POINT('',(-0.05,-1.3,-0.5));
#7913=CARTESIAN_POINT('Ctrl Pts',(-0.05,1.19895788082818,-0.5));
#7914=CARTESIAN_POINT('Ctrl Pts',(-0.05,1.19895788082818,-0.506278891478307));
#7915=CARTESIAN_POINT('Ctrl Pts',(-0.0487450133099082,1.19901227819454,
-0.512975804624065));
#7916=CARTESIAN_POINT('Ctrl Pts',(-0.0436421041657015,1.19920885850753,
-0.52529455629072));
#7917=CARTESIAN_POINT('Ctrl Pts',(-0.0397942217705327,1.1993482149535,-0.530916456348121));
#7918=CARTESIAN_POINT('Ctrl Pts',(-0.0309164568000038,1.19960989221221,
-0.539794221318651));
#7919=CARTESIAN_POINT('Ctrl Pts',(-0.0252945565319676,1.19974919586288,
-0.543642104041954));
#7920=CARTESIAN_POINT('Ctrl Pts',(-0.0129758042228731,1.19994565546462,
-0.548745013499911));
#7921=CARTESIAN_POINT('Ctrl Pts',(-0.0062788908391104,1.2,-0.55));
#7922=CARTESIAN_POINT('Ctrl Pts',(0.00627889083911043,1.2,-0.55));
#7923=CARTESIAN_POINT('Ctrl Pts',(0.0129758042228731,1.19994565546462,-0.548745013499911));
#7924=CARTESIAN_POINT('Ctrl Pts',(0.0252945565319676,1.19974919586288,-0.543642104041954));
#7925=CARTESIAN_POINT('Ctrl Pts',(0.0309164568000038,1.19960989221221,-0.539794221318651));
#7926=CARTESIAN_POINT('Ctrl Pts',(0.0397942217705327,1.1993482149535,-0.530916456348121));
#7927=CARTESIAN_POINT('Ctrl Pts',(0.0436421041657015,1.19920885850753,-0.52529455629072));
#7928=CARTESIAN_POINT('Ctrl Pts',(0.0487450133099082,1.19901227819454,-0.512975804624065));
#7929=CARTESIAN_POINT('Ctrl Pts',(0.05,1.19895788082818,-0.506278891478307));
#7930=CARTESIAN_POINT('Ctrl Pts',(0.05,1.19895788082818,-0.493721108521693));
#7931=CARTESIAN_POINT('Ctrl Pts',(0.0487450133099082,1.19901227819454,-0.487024195375935));
#7932=CARTESIAN_POINT('Ctrl Pts',(0.0436421041657013,1.19920885850753,-0.47470544370928));
#7933=CARTESIAN_POINT('Ctrl Pts',(0.0397942217705328,1.1993482149535,-0.469083543651878));
#7934=CARTESIAN_POINT('Ctrl Pts',(0.0309164568000038,1.19960989221221,-0.460205778681349));
#7935=CARTESIAN_POINT('Ctrl Pts',(0.0252945565319674,1.19974919586288,-0.456357895958046));
#7936=CARTESIAN_POINT('Ctrl Pts',(0.012975804222873,1.19994565546462,-0.451254986500089));
#7937=CARTESIAN_POINT('Ctrl Pts',(0.00627889083911038,1.2,-0.45));
#7938=CARTESIAN_POINT('Ctrl Pts',(-0.00627889083911039,1.2,-0.45));
#7939=CARTESIAN_POINT('Ctrl Pts',(-0.012975804222873,1.19994565546462,-0.451254986500089));
#7940=CARTESIAN_POINT('Ctrl Pts',(-0.0252945565319674,1.19974919586288,
-0.456357895958046));
#7941=CARTESIAN_POINT('Ctrl Pts',(-0.0309164568000038,1.19960989221221,
-0.460205778681349));
#7942=CARTESIAN_POINT('Ctrl Pts',(-0.0397942217705328,1.1993482149535,-0.469083543651878));
#7943=CARTESIAN_POINT('Ctrl Pts',(-0.0436421041657013,1.19920885850753,
-0.47470544370928));
#7944=CARTESIAN_POINT('Ctrl Pts',(-0.0487450133099082,1.19901227819454,
-0.487024195375935));
#7945=CARTESIAN_POINT('Ctrl Pts',(-0.05,1.19895788082818,-0.493721108521693));
#7946=CARTESIAN_POINT('Ctrl Pts',(-0.05,1.19895788082818,-0.5));
#7947=CARTESIAN_POINT('Origin',(-1.3,0.,-2.5));
#7948=CARTESIAN_POINT('',(-1.19895788082818,0.0499999999999998,-2.5));
#7949=CARTESIAN_POINT('',(-1.2,-6.12323399573674E-18,-2.45));
#7950=CARTESIAN_POINT('Ctrl Pts',(-1.19895788082818,0.0499999999999998,
-2.5));
#7951=CARTESIAN_POINT('Ctrl Pts',(-1.19895788082818,0.0499999999999998,
-2.49372110852169));
#7952=CARTESIAN_POINT('Ctrl Pts',(-1.19901227819454,0.0487450133099079,
-2.48702419537593));
#7953=CARTESIAN_POINT('Ctrl Pts',(-1.19920885850753,0.0436421041657012,
-2.47470544370928));
#7954=CARTESIAN_POINT('Ctrl Pts',(-1.1993482149535,0.0397942217705327,-2.46908354365188));
#7955=CARTESIAN_POINT('Ctrl Pts',(-1.19960989221221,0.0309164568000037,
-2.46020577868135));
#7956=CARTESIAN_POINT('Ctrl Pts',(-1.19974919586288,0.0252945565319673,
-2.45635789595805));
#7957=CARTESIAN_POINT('Ctrl Pts',(-1.19994565546462,0.0129758042228729,
-2.45125498650009));
#7958=CARTESIAN_POINT('Ctrl Pts',(-1.2,0.00627889083911036,-2.45));
#7959=CARTESIAN_POINT('Ctrl Pts',(-1.2,6.07153216591882E-18,-2.45));
#7960=CARTESIAN_POINT('',(-1.2,-7.88998188112687E-17,-2.55));
#7961=CARTESIAN_POINT('Ctrl Pts',(-1.2,-1.0842021724855E-17,-2.55));
#7962=CARTESIAN_POINT('Ctrl Pts',(-1.2,0.00627889083911035,-2.55));
#7963=CARTESIAN_POINT('Ctrl Pts',(-1.19994565546462,0.0129758042228729,
-2.54874501349991));
#7964=CARTESIAN_POINT('Ctrl Pts',(-1.19974919586288,0.0252945565319673,
-2.54364210404195));
#7965=CARTESIAN_POINT('Ctrl Pts',(-1.19960989221221,0.0309164568000037,
-2.53979422131865));
#7966=CARTESIAN_POINT('Ctrl Pts',(-1.1993482149535,0.0397942217705327,-2.53091645634812));
#7967=CARTESIAN_POINT('Ctrl Pts',(-1.19920885850753,0.0436421041657012,
-2.52529455629072));
#7968=CARTESIAN_POINT('Ctrl Pts',(-1.19901227819454,0.0487450133099079,
-2.51297580462407));
#7969=CARTESIAN_POINT('Ctrl Pts',(-1.19895788082818,0.0499999999999998,
-2.50627889147831));
#7970=CARTESIAN_POINT('Ctrl Pts',(-1.19895788082818,0.0499999999999998,
-2.5));
#7971=CARTESIAN_POINT('Ctrl Pts',(-1.2,6.07153216591882E-18,-2.45));
#7972=CARTESIAN_POINT('Ctrl Pts',(-1.2,-0.00627889083911035,-2.45));
#7973=CARTESIAN_POINT('Ctrl Pts',(-1.19994565546462,-0.0129758042228729,
-2.45125498650009));
#7974=CARTESIAN_POINT('Ctrl Pts',(-1.19974919586288,-0.0252945565319673,
-2.45635789595805));
#7975=CARTESIAN_POINT('Ctrl Pts',(-1.19960989221221,-0.0309164568000037,
-2.46020577868135));
#7976=CARTESIAN_POINT('Ctrl Pts',(-1.1993482149535,-0.0397942217705327,
-2.46908354365188));
#7977=CARTESIAN_POINT('Ctrl Pts',(-1.19920885850753,-0.0436421041657012,
-2.47470544370928));
#7978=CARTESIAN_POINT('Ctrl Pts',(-1.19901227819454,-0.0487450133099079,
-2.48702419537593));
#7979=CARTESIAN_POINT('Ctrl Pts',(-1.19895788082818,-0.0499999999999998,
-2.49372110852169));
#7980=CARTESIAN_POINT('Ctrl Pts',(-1.19895788082818,-0.0499999999999998,
-2.50627889147831));
#7981=CARTESIAN_POINT('Ctrl Pts',(-1.19901227819454,-0.0487450133099079,
-2.51297580462407));
#7982=CARTESIAN_POINT('Ctrl Pts',(-1.19920885850753,-0.0436421041657012,
-2.52529455629072));
#7983=CARTESIAN_POINT('Ctrl Pts',(-1.1993482149535,-0.0397942217705327,
-2.53091645634812));
#7984=CARTESIAN_POINT('Ctrl Pts',(-1.19960989221221,-0.0309164568000037,
-2.53979422131865));
#7985=CARTESIAN_POINT('Ctrl Pts',(-1.19974919586288,-0.0252945565319673,
-2.54364210404195));
#7986=CARTESIAN_POINT('Ctrl Pts',(-1.19994565546462,-0.0129758042228729,
-2.54874501349991));
#7987=CARTESIAN_POINT('Ctrl Pts',(-1.2,-0.00627889083911037,-2.55));
#7988=CARTESIAN_POINT('Ctrl Pts',(-1.2,-1.0842021724855E-17,-2.55));
#7989=CARTESIAN_POINT('',(-0.4,-6.53106394982199E-18,-2.45));
#7990=CARTESIAN_POINT('',(-1.3,-6.12323399573674E-18,-2.45));
#7991=CARTESIAN_POINT('',(-0.4,-2.44929359829471E-17,-2.55));
#7992=CARTESIAN_POINT('Ctrl Pts',(-0.4,0.,-2.55));
#7993=CARTESIAN_POINT('Ctrl Pts',(-0.4,-0.00628514845714645,-2.55));
#7994=CARTESIAN_POINT('Ctrl Pts',(-0.399836729543542,-0.0129847676279312,
-2.5487425667586));
#7995=CARTESIAN_POINT('Ctrl Pts',(-0.399246581249293,-0.0253018150396575,
-2.5436378293633));
#7996=CARTESIAN_POINT('Ctrl Pts',(-0.398828027526425,-0.0309197907817456,
-2.53979088733691));
#7997=CARTESIAN_POINT('Ctrl Pts',(-0.398040841710914,-0.0397909243921695,
-2.53091975372649));
#7998=CARTESIAN_POINT('Ctrl Pts',(-0.397620851691571,-0.0436378373878614,
-2.52530179409386));
#7999=CARTESIAN_POINT('Ctrl Pts',(-0.397027412247524,-0.0487425534891113,
-2.51298480122901));
#8000=CARTESIAN_POINT('Ctrl Pts',(-0.396862696659689,-0.0499999999999998,
-2.50628520096426));
#8001=CARTESIAN_POINT('Ctrl Pts',(-0.396862696659689,-0.0499999999999998,
-2.49371479903574));
#8002=CARTESIAN_POINT('Ctrl Pts',(-0.397027412247524,-0.0487425534891114,
-2.48701519877099));
#8003=CARTESIAN_POINT('Ctrl Pts',(-0.397620851691571,-0.0436378373878616,
-2.47469820590614));
#8004=CARTESIAN_POINT('Ctrl Pts',(-0.398040841710914,-0.0397909243921695,
-2.46908024627351));
#8005=CARTESIAN_POINT('Ctrl Pts',(-0.398828027526425,-0.0309197907817457,
-2.46020911266309));
#8006=CARTESIAN_POINT('Ctrl Pts',(-0.399246581249293,-0.0253018150396575,
-2.4563621706367));
#8007=CARTESIAN_POINT('Ctrl Pts',(-0.399836729543542,-0.0129847676279312,
-2.4512574332414));
#8008=CARTESIAN_POINT('Ctrl Pts',(-0.4,-0.00628514845714645,-2.45));
#8009=CARTESIAN_POINT('Ctrl Pts',(-0.4,-6.93889390390723E-18,-2.45));
#8010=CARTESIAN_POINT('',(-0.396862696659689,0.0499999999999998,-2.5));
#8011=CARTESIAN_POINT('Ctrl Pts',(-0.396862696659689,0.0499999999999998,
-2.5));
#8012=CARTESIAN_POINT('Ctrl Pts',(-0.396862696659689,0.0499999999999998,
-2.50628520096426));
#8013=CARTESIAN_POINT('Ctrl Pts',(-0.397027412247524,0.0487425534891114,
-2.51298480122901));
#8014=CARTESIAN_POINT('Ctrl Pts',(-0.397620851691571,0.0436378373878616,
-2.52530179409386));
#8015=CARTESIAN_POINT('Ctrl Pts',(-0.398040841710914,0.0397909243921695,
-2.53091975372649));
#8016=CARTESIAN_POINT('Ctrl Pts',(-0.398828027526425,0.0309197907817456,
-2.53979088733691));
#8017=CARTESIAN_POINT('Ctrl Pts',(-0.399246581249293,0.0253018150396575,
-2.5436378293633));
#8018=CARTESIAN_POINT('Ctrl Pts',(-0.399836729543542,0.0129847676279312,
-2.5487425667586));
#8019=CARTESIAN_POINT('Ctrl Pts',(-0.4,0.00628514845714645,-2.55));
#8020=CARTESIAN_POINT('Ctrl Pts',(-0.4,0.,-2.55));
#8021=CARTESIAN_POINT('Ctrl Pts',(-0.4,-6.93889390390723E-18,-2.45));
#8022=CARTESIAN_POINT('Ctrl Pts',(-0.4,0.00628514845714644,-2.45));
#8023=CARTESIAN_POINT('Ctrl Pts',(-0.399836729543542,0.0129847676279312,
-2.4512574332414));
#8024=CARTESIAN_POINT('Ctrl Pts',(-0.399246581249293,0.0253018150396575,
-2.4563621706367));
#8025=CARTESIAN_POINT('Ctrl Pts',(-0.398828027526425,0.0309197907817456,
-2.46020911266309));
#8026=CARTESIAN_POINT('Ctrl Pts',(-0.398040841710914,0.0397909243921695,
-2.46908024627351));
#8027=CARTESIAN_POINT('Ctrl Pts',(-0.397620851691571,0.0436378373878614,
-2.47469820590614));
#8028=CARTESIAN_POINT('Ctrl Pts',(-0.397027412247524,0.0487425534891113,
-2.48701519877099));
#8029=CARTESIAN_POINT('Ctrl Pts',(-0.396862696659689,0.0499999999999998,
-2.49371479903574));
#8030=CARTESIAN_POINT('Ctrl Pts',(-0.396862696659689,0.0499999999999998,
-2.5));
#8031=CARTESIAN_POINT('Origin',(-1.3,0.,-2.5));
#8032=CARTESIAN_POINT('',(0.396862696659689,0.0499999999999998,-2.5));
#8033=CARTESIAN_POINT('',(0.4,-6.74790438431909E-18,-2.45));
#8034=CARTESIAN_POINT('Ctrl Pts',(0.396862696659689,0.0499999999999998,
-2.5));
#8035=CARTESIAN_POINT('Ctrl Pts',(0.396862696659689,0.0499999999999998,
-2.49371479903574));
#8036=CARTESIAN_POINT('Ctrl Pts',(0.397027412247524,0.0487425534891114,
-2.48701519877099));
#8037=CARTESIAN_POINT('Ctrl Pts',(0.397620851691571,0.0436378373878616,
-2.47469820590614));
#8038=CARTESIAN_POINT('Ctrl Pts',(0.398040841710914,0.0397909243921695,
-2.46908024627351));
#8039=CARTESIAN_POINT('Ctrl Pts',(0.398828027526425,0.0309197907817456,
-2.46020911266309));
#8040=CARTESIAN_POINT('Ctrl Pts',(0.399246581249293,0.0253018150396575,
-2.4563621706367));
#8041=CARTESIAN_POINT('Ctrl Pts',(0.399836729543542,0.0129847676279312,
-2.4512574332414));
#8042=CARTESIAN_POINT('Ctrl Pts',(0.4,0.00628514845714644,-2.45));
#8043=CARTESIAN_POINT('Ctrl Pts',(0.4,-7.37257477290143E-18,-2.45));
#8044=CARTESIAN_POINT('Ctrl Pts',(0.4,-7.37257477290143E-18,-2.45));
#8045=CARTESIAN_POINT('Ctrl Pts',(0.4,-0.00628514845714645,-2.45));
#8046=CARTESIAN_POINT('Ctrl Pts',(0.399836729543542,-0.0129847676279312,
-2.4512574332414));
#8047=CARTESIAN_POINT('Ctrl Pts',(0.399246581249293,-0.0253018150396575,
-2.4563621706367));
#8048=CARTESIAN_POINT('Ctrl Pts',(0.398828027526425,-0.0309197907817457,
-2.46020911266309));
#8049=CARTESIAN_POINT('Ctrl Pts',(0.398040841710914,-0.0397909243921695,
-2.46908024627351));
#8050=CARTESIAN_POINT('Ctrl Pts',(0.397620851691571,-0.0436378373878616,
-2.47469820590614));
#8051=CARTESIAN_POINT('Ctrl Pts',(0.397027412247524,-0.0487425534891114,
-2.48701519877099));
#8052=CARTESIAN_POINT('Ctrl Pts',(0.396862696659689,-0.0499999999999998,
-2.49371479903574));
#8053=CARTESIAN_POINT('Ctrl Pts',(0.396862696659689,-0.0499999999999998,
-2.50628520096426));
#8054=CARTESIAN_POINT('Ctrl Pts',(0.397027412247524,-0.0487425534891113,
-2.51298480122901));
#8055=CARTESIAN_POINT('Ctrl Pts',(0.397620851691571,-0.0436378373878614,
-2.52530179409386));
#8056=CARTESIAN_POINT('Ctrl Pts',(0.398040841710914,-0.0397909243921695,
-2.53091975372649));
#8057=CARTESIAN_POINT('Ctrl Pts',(0.398828027526425,-0.0309197907817457,
-2.53979088733691));
#8058=CARTESIAN_POINT('Ctrl Pts',(0.399246581249293,-0.0253018150396572,
-2.5436378293633));
#8059=CARTESIAN_POINT('Ctrl Pts',(0.399836729543542,-0.0129847676279309,
-2.5487425667586));
#8060=CARTESIAN_POINT('Ctrl Pts',(0.4,-0.00628514845714645,-2.55));
#8061=CARTESIAN_POINT('Ctrl Pts',(0.4,0.00628514845714645,-2.55));
#8062=CARTESIAN_POINT('Ctrl Pts',(0.399836729543542,0.0129847676279312,
-2.5487425667586));
#8063=CARTESIAN_POINT('Ctrl Pts',(0.399246581249293,0.0253018150396575,
-2.5436378293633));
#8064=CARTESIAN_POINT('Ctrl Pts',(0.398828027526425,0.0309197907817456,
-2.53979088733691));
#8065=CARTESIAN_POINT('Ctrl Pts',(0.398040841710914,0.0397909243921695,
-2.53091975372649));
#8066=CARTESIAN_POINT('Ctrl Pts',(0.397620851691571,0.0436378373878616,
-2.52530179409386));
#8067=CARTESIAN_POINT('Ctrl Pts',(0.397027412247524,0.0487425534891114,
-2.51298480122901));
#8068=CARTESIAN_POINT('Ctrl Pts',(0.396862696659689,0.0499999999999998,
-2.50628520096426));
#8069=CARTESIAN_POINT('Ctrl Pts',(0.396862696659689,0.0499999999999998,
-2.5));
#8070=CARTESIAN_POINT('',(1.2,-6.12323399573674E-18,-2.45));
#8071=CARTESIAN_POINT('',(-1.3,-6.12323399573674E-18,-2.45));
#8072=CARTESIAN_POINT('',(1.19895788082818,0.0499999999999998,-2.5));
#8073=CARTESIAN_POINT('Ctrl Pts',(1.19895788082818,0.0499999999999998,-2.5));
#8074=CARTESIAN_POINT('Ctrl Pts',(1.19895788082818,0.0499999999999998,-2.50627889147831));
#8075=CARTESIAN_POINT('Ctrl Pts',(1.19901227819454,0.0487450133099079,-2.51297580462407));
#8076=CARTESIAN_POINT('Ctrl Pts',(1.19920885850753,0.0436421041657012,-2.52529455629072));
#8077=CARTESIAN_POINT('Ctrl Pts',(1.1993482149535,0.0397942217705327,-2.53091645634812));
#8078=CARTESIAN_POINT('Ctrl Pts',(1.19960989221221,0.0309164568000037,-2.53979422131865));
#8079=CARTESIAN_POINT('Ctrl Pts',(1.19974919586288,0.0252945565319673,-2.54364210404195));
#8080=CARTESIAN_POINT('Ctrl Pts',(1.19994565546462,0.0129758042228729,-2.54874501349991));
#8081=CARTESIAN_POINT('Ctrl Pts',(1.2,0.00627889083911035,-2.55));
#8082=CARTESIAN_POINT('Ctrl Pts',(1.2,-0.00627889083911037,-2.55));
#8083=CARTESIAN_POINT('Ctrl Pts',(1.19994565546462,-0.0129758042228729,
-2.54874501349991));
#8084=CARTESIAN_POINT('Ctrl Pts',(1.19974919586288,-0.0252945565319673,
-2.54364210404195));
#8085=CARTESIAN_POINT('Ctrl Pts',(1.19960989221221,-0.0309164568000037,
-2.53979422131865));
#8086=CARTESIAN_POINT('Ctrl Pts',(1.1993482149535,-0.0397942217705327,-2.53091645634812));
#8087=CARTESIAN_POINT('Ctrl Pts',(1.19920885850753,-0.0436421041657012,
-2.52529455629072));
#8088=CARTESIAN_POINT('Ctrl Pts',(1.19901227819454,-0.0487450133099079,
-2.51297580462407));
#8089=CARTESIAN_POINT('Ctrl Pts',(1.19895788082818,-0.0499999999999998,
-2.50627889147831));
#8090=CARTESIAN_POINT('Ctrl Pts',(1.19895788082818,-0.0499999999999998,
-2.49372110852169));
#8091=CARTESIAN_POINT('Ctrl Pts',(1.19901227819454,-0.0487450133099081,
-2.48702419537594));
#8092=CARTESIAN_POINT('Ctrl Pts',(1.19920885850753,-0.0436421041657014,
-2.47470544370928));
#8093=CARTESIAN_POINT('Ctrl Pts',(1.1993482149535,-0.0397942217705327,-2.46908354365188));
#8094=CARTESIAN_POINT('Ctrl Pts',(1.19960989221221,-0.0309164568000037,
-2.46020577868135));
#8095=CARTESIAN_POINT('Ctrl Pts',(1.19974919586288,-0.0252945565319673,
-2.45635789595805));
#8096=CARTESIAN_POINT('Ctrl Pts',(1.19994565546462,-0.0129758042228729,
-2.45125498650009));
#8097=CARTESIAN_POINT('Ctrl Pts',(1.2,-0.00627889083911035,-2.45));
#8098=CARTESIAN_POINT('Ctrl Pts',(1.2,6.07153216591882E-18,-2.45));
#8099=CARTESIAN_POINT('Ctrl Pts',(1.2,6.07153216591882E-18,-2.45));
#8100=CARTESIAN_POINT('Ctrl Pts',(1.2,0.00627889083911036,-2.45));
#8101=CARTESIAN_POINT('Ctrl Pts',(1.19994565546462,0.0129758042228729,-2.45125498650009));
#8102=CARTESIAN_POINT('Ctrl Pts',(1.19974919586288,0.0252945565319673,-2.45635789595805));
#8103=CARTESIAN_POINT('Ctrl Pts',(1.19960989221221,0.0309164568000037,-2.46020577868135));
#8104=CARTESIAN_POINT('Ctrl Pts',(1.1993482149535,0.0397942217705327,-2.46908354365188));
#8105=CARTESIAN_POINT('Ctrl Pts',(1.19920885850753,0.0436421041657012,-2.47470544370928));
#8106=CARTESIAN_POINT('Ctrl Pts',(1.19901227819454,0.0487450133099079,-2.48702419537593));
#8107=CARTESIAN_POINT('Ctrl Pts',(1.19895788082818,0.0499999999999998,-2.49372110852169));
#8108=CARTESIAN_POINT('Ctrl Pts',(1.19895788082818,0.0499999999999998,-2.5));
#8109=CARTESIAN_POINT('Origin',(-1.3,0.,-1.5));
#8110=CARTESIAN_POINT('',(-1.19895788082818,0.05,-1.5));
#8111=CARTESIAN_POINT('',(-1.2,-6.12323399573677E-18,-1.45));
#8112=CARTESIAN_POINT('Ctrl Pts',(-1.19895788082818,0.05,-1.5));
#8113=CARTESIAN_POINT('Ctrl Pts',(-1.19895788082818,0.05,-1.49372110852169));
#8114=CARTESIAN_POINT('Ctrl Pts',(-1.19901227819454,0.0487450133099082,
-1.48702419537594));
#8115=CARTESIAN_POINT('Ctrl Pts',(-1.19920885850753,0.0436421041657014,
-1.47470544370928));
#8116=CARTESIAN_POINT('Ctrl Pts',(-1.1993482149535,0.0397942217705329,-1.46908354365188));
#8117=CARTESIAN_POINT('Ctrl Pts',(-1.19960989221221,0.0309164568000038,
-1.46020577868135));
#8118=CARTESIAN_POINT('Ctrl Pts',(-1.19974919586288,0.0252945565319674,
-1.45635789595805));
#8119=CARTESIAN_POINT('Ctrl Pts',(-1.19994565546462,0.012975804222873,-1.45125498650009));
#8120=CARTESIAN_POINT('Ctrl Pts',(-1.2,0.00627889083911039,-1.45));
#8121=CARTESIAN_POINT('Ctrl Pts',(-1.2,7.37257477290143E-18,-1.45));
#8122=CARTESIAN_POINT('',(-1.2,-7.84661379422745E-17,-1.55));
#8123=CARTESIAN_POINT('Ctrl Pts',(-1.2,-9.97465998686664E-18,-1.55));
#8124=CARTESIAN_POINT('Ctrl Pts',(-1.2,0.00627889083911038,-1.55));
#8125=CARTESIAN_POINT('Ctrl Pts',(-1.19994565546462,0.0129758042228729,
-1.54874501349991));
#8126=CARTESIAN_POINT('Ctrl Pts',(-1.19974919586288,0.0252945565319674,
-1.54364210404195));
#8127=CARTESIAN_POINT('Ctrl Pts',(-1.19960989221221,0.0309164568000038,
-1.53979422131865));
#8128=CARTESIAN_POINT('Ctrl Pts',(-1.1993482149535,0.0397942217705328,-1.53091645634812));
#8129=CARTESIAN_POINT('Ctrl Pts',(-1.19920885850753,0.0436421041657013,
-1.52529455629072));
#8130=CARTESIAN_POINT('Ctrl Pts',(-1.19901227819454,0.0487450133099081,
-1.51297580462407));
#8131=CARTESIAN_POINT('Ctrl Pts',(-1.19895788082818,0.05,-1.50627889147831));
#8132=CARTESIAN_POINT('Ctrl Pts',(-1.19895788082818,0.05,-1.5));
#8133=CARTESIAN_POINT('Ctrl Pts',(-1.2,7.37257477290143E-18,-1.45));
#8134=CARTESIAN_POINT('Ctrl Pts',(-1.2,-0.00627889083911038,-1.45));
#8135=CARTESIAN_POINT('Ctrl Pts',(-1.19994565546462,-0.0129758042228731,
-1.45125498650009));
#8136=CARTESIAN_POINT('Ctrl Pts',(-1.19974919586288,-0.0252945565319675,
-1.45635789595805));
#8137=CARTESIAN_POINT('Ctrl Pts',(-1.19960989221221,-0.0309164568000038,
-1.46020577868135));
#8138=CARTESIAN_POINT('Ctrl Pts',(-1.1993482149535,-0.0397942217705328,
-1.46908354365188));
#8139=CARTESIAN_POINT('Ctrl Pts',(-1.19920885850753,-0.0436421041657014,
-1.47470544370928));
#8140=CARTESIAN_POINT('Ctrl Pts',(-1.19901227819454,-0.0487450133099082,
-1.48702419537594));
#8141=CARTESIAN_POINT('Ctrl Pts',(-1.19895788082818,-0.05,-1.49372110852169));
#8142=CARTESIAN_POINT('Ctrl Pts',(-1.19895788082818,-0.05,-1.50627889147831));
#8143=CARTESIAN_POINT('Ctrl Pts',(-1.19901227819454,-0.0487450133099082,
-1.51297580462406));
#8144=CARTESIAN_POINT('Ctrl Pts',(-1.19920885850753,-0.0436421041657014,
-1.52529455629072));
#8145=CARTESIAN_POINT('Ctrl Pts',(-1.1993482149535,-0.0397942217705328,
-1.53091645634812));
#8146=CARTESIAN_POINT('Ctrl Pts',(-1.19960989221221,-0.0309164568000038,
-1.53979422131865));
#8147=CARTESIAN_POINT('Ctrl Pts',(-1.19974919586288,-0.0252945565319672,
-1.54364210404195));
#8148=CARTESIAN_POINT('Ctrl Pts',(-1.19994565546462,-0.0129758042228727,
-1.54874501349991));
#8149=CARTESIAN_POINT('Ctrl Pts',(-1.2,-0.0062788908391104,-1.55));
#8150=CARTESIAN_POINT('Ctrl Pts',(-1.2,-9.97465998686664E-18,-1.55));
#8151=CARTESIAN_POINT('',(-0.4,-6.0973830808278E-18,-1.45));
#8152=CARTESIAN_POINT('',(-1.3,-6.12323399573677E-18,-1.45));
#8153=CARTESIAN_POINT('',(-0.4,-2.427609554845E-17,-1.55));
#8154=CARTESIAN_POINT('Ctrl Pts',(-0.4,4.33680868994202E-19,-1.55));
#8155=CARTESIAN_POINT('Ctrl Pts',(-0.4,-0.00628514845714649,-1.55));
#8156=CARTESIAN_POINT('Ctrl Pts',(-0.399836729543542,-0.0129847676279311,
-1.5487425667586));
#8157=CARTESIAN_POINT('Ctrl Pts',(-0.399246581249293,-0.0253018150396574,
-1.5436378293633));
#8158=CARTESIAN_POINT('Ctrl Pts',(-0.398828027526425,-0.0309197907817458,
-1.53979088733691));
#8159=CARTESIAN_POINT('Ctrl Pts',(-0.398040841710914,-0.0397909243921696,
-1.53091975372649));
#8160=CARTESIAN_POINT('Ctrl Pts',(-0.397620851691571,-0.0436378373878618,
-1.52530179409386));
#8161=CARTESIAN_POINT('Ctrl Pts',(-0.397027412247524,-0.0487425534891115,
-1.51298480122901));
#8162=CARTESIAN_POINT('Ctrl Pts',(-0.396862696659689,-0.05,-1.50628520096426));
#8163=CARTESIAN_POINT('Ctrl Pts',(-0.396862696659689,-0.05,-1.49371479903575));
#8164=CARTESIAN_POINT('Ctrl Pts',(-0.397027412247524,-0.0487425534891117,
-1.48701519877099));
#8165=CARTESIAN_POINT('Ctrl Pts',(-0.397620851691571,-0.0436378373878621,
-1.47469820590614));
#8166=CARTESIAN_POINT('Ctrl Pts',(-0.398040841710914,-0.0397909243921697,
-1.46908024627352));
#8167=CARTESIAN_POINT('Ctrl Pts',(-0.398828027526425,-0.0309197907817458,
-1.46020911266309));
#8168=CARTESIAN_POINT('Ctrl Pts',(-0.399246581249293,-0.0253018150396577,
-1.4563621706367));
#8169=CARTESIAN_POINT('Ctrl Pts',(-0.399836729543542,-0.0129847676279314,
-1.4512574332414));
#8170=CARTESIAN_POINT('Ctrl Pts',(-0.4,-0.00628514845714648,-1.45));
#8171=CARTESIAN_POINT('Ctrl Pts',(-0.4,-6.07153216591882E-18,-1.45));
#8172=CARTESIAN_POINT('',(-0.396862696659689,0.05,-1.5));
#8173=CARTESIAN_POINT('Ctrl Pts',(-0.396862696659689,0.05,-1.5));
#8174=CARTESIAN_POINT('Ctrl Pts',(-0.396862696659689,0.05,-1.50628520096425));
#8175=CARTESIAN_POINT('Ctrl Pts',(-0.397027412247524,0.0487425534891116,
-1.51298480122901));
#8176=CARTESIAN_POINT('Ctrl Pts',(-0.397620851691571,0.0436378373878619,
-1.52530179409386));
#8177=CARTESIAN_POINT('Ctrl Pts',(-0.398040841710914,0.0397909243921696,
-1.53091975372649));
#8178=CARTESIAN_POINT('Ctrl Pts',(-0.398828027526425,0.0309197907817458,
-1.53979088733691));
#8179=CARTESIAN_POINT('Ctrl Pts',(-0.399246581249293,0.0253018150396575,
-1.5436378293633));
#8180=CARTESIAN_POINT('Ctrl Pts',(-0.399836729543542,0.0129847676279312,
-1.54874256675859));
#8181=CARTESIAN_POINT('Ctrl Pts',(-0.4,0.00628514845714648,-1.55));
#8182=CARTESIAN_POINT('Ctrl Pts',(-0.4,4.33680868994202E-19,-1.55));
#8183=CARTESIAN_POINT('Ctrl Pts',(-0.4,-6.07153216591882E-18,-1.45));
#8184=CARTESIAN_POINT('Ctrl Pts',(-0.4,0.00628514845714647,-1.45));
#8185=CARTESIAN_POINT('Ctrl Pts',(-0.399836729543542,0.0129847676279314,
-1.45125743324141));
#8186=CARTESIAN_POINT('Ctrl Pts',(-0.399246581249293,0.0253018150396577,
-1.4563621706367));
#8187=CARTESIAN_POINT('Ctrl Pts',(-0.398828027526425,0.0309197907817458,
-1.46020911266309));
#8188=CARTESIAN_POINT('Ctrl Pts',(-0.398040841710914,0.0397909243921697,
-1.46908024627351));
#8189=CARTESIAN_POINT('Ctrl Pts',(-0.397620851691571,0.0436378373878618,
-1.47469820590614));
#8190=CARTESIAN_POINT('Ctrl Pts',(-0.397027412247524,0.0487425534891115,
-1.48701519877099));
#8191=CARTESIAN_POINT('Ctrl Pts',(-0.396862696659689,0.05,-1.49371479903574));
#8192=CARTESIAN_POINT('Ctrl Pts',(-0.396862696659689,0.05,-1.5));
#8193=CARTESIAN_POINT('Origin',(-1.3,0.,-1.5));
#8194=CARTESIAN_POINT('',(0.396862696659689,0.05,-1.5));
#8195=CARTESIAN_POINT('',(0.4,-6.3142235153249E-18,-1.45));
#8196=CARTESIAN_POINT('Ctrl Pts',(0.396862696659689,0.05,-1.5));
#8197=CARTESIAN_POINT('Ctrl Pts',(0.396862696659689,0.05,-1.49371479903575));
#8198=CARTESIAN_POINT('Ctrl Pts',(0.397027412247524,0.0487425534891116,
-1.48701519877099));
#8199=CARTESIAN_POINT('Ctrl Pts',(0.397620851691571,0.0436378373878619,
-1.47469820590614));
#8200=CARTESIAN_POINT('Ctrl Pts',(0.398040841710914,0.0397909243921697,
-1.46908024627351));
#8201=CARTESIAN_POINT('Ctrl Pts',(0.398828027526425,0.0309197907817458,
-1.46020911266309));
#8202=CARTESIAN_POINT('Ctrl Pts',(0.399246581249293,0.0253018150396577,
-1.4563621706367));
#8203=CARTESIAN_POINT('Ctrl Pts',(0.399836729543542,0.0129847676279313,
-1.4512574332414));
#8204=CARTESIAN_POINT('Ctrl Pts',(0.4,0.00628514845714647,-1.45));
#8205=CARTESIAN_POINT('Ctrl Pts',(0.4,-6.50521303491303E-18,-1.45));
#8206=CARTESIAN_POINT('Ctrl Pts',(0.4,-6.50521303491303E-18,-1.45));
#8207=CARTESIAN_POINT('Ctrl Pts',(0.4,-0.00628514845714648,-1.45));
#8208=CARTESIAN_POINT('Ctrl Pts',(0.399836729543542,-0.0129847676279314,
-1.4512574332414));
#8209=CARTESIAN_POINT('Ctrl Pts',(0.399246581249293,-0.0253018150396577,
-1.4563621706367));
#8210=CARTESIAN_POINT('Ctrl Pts',(0.398828027526425,-0.0309197907817458,
-1.46020911266309));
#8211=CARTESIAN_POINT('Ctrl Pts',(0.398040841710914,-0.0397909243921697,
-1.46908024627351));
#8212=CARTESIAN_POINT('Ctrl Pts',(0.397620851691571,-0.0436378373878622,
-1.47469820590614));
#8213=CARTESIAN_POINT('Ctrl Pts',(0.397027412247524,-0.0487425534891117,
-1.48701519877099));
#8214=CARTESIAN_POINT('Ctrl Pts',(0.396862696659689,-0.05,-1.49371479903575));
#8215=CARTESIAN_POINT('Ctrl Pts',(0.396862696659689,-0.05,-1.50628520096425));
#8216=CARTESIAN_POINT('Ctrl Pts',(0.397027412247524,-0.0487425534891116,
-1.51298480122901));
#8217=CARTESIAN_POINT('Ctrl Pts',(0.397620851691571,-0.0436378373878619,
-1.52530179409386));
#8218=CARTESIAN_POINT('Ctrl Pts',(0.398040841710914,-0.0397909243921696,
-1.53091975372649));
#8219=CARTESIAN_POINT('Ctrl Pts',(0.398828027526425,-0.0309197907817458,
-1.53979088733691));
#8220=CARTESIAN_POINT('Ctrl Pts',(0.399246581249293,-0.0253018150396575,
-1.5436378293633));
#8221=CARTESIAN_POINT('Ctrl Pts',(0.399836729543542,-0.0129847676279312,
-1.54874256675859));
#8222=CARTESIAN_POINT('Ctrl Pts',(0.4,-0.00628514845714648,-1.55));
#8223=CARTESIAN_POINT('Ctrl Pts',(0.4,0.00628514845714648,-1.55));
#8224=CARTESIAN_POINT('Ctrl Pts',(0.399836729543542,0.0129847676279312,
-1.54874256675859));
#8225=CARTESIAN_POINT('Ctrl Pts',(0.399246581249293,0.0253018150396575,
-1.5436378293633));
#8226=CARTESIAN_POINT('Ctrl Pts',(0.398828027526425,0.0309197907817458,
-1.53979088733691));
#8227=CARTESIAN_POINT('Ctrl Pts',(0.398040841710914,0.0397909243921696,
-1.53091975372649));
#8228=CARTESIAN_POINT('Ctrl Pts',(0.397620851691571,0.0436378373878622,
-1.52530179409386));
#8229=CARTESIAN_POINT('Ctrl Pts',(0.397027412247524,0.0487425534891117,
-1.51298480122901));
#8230=CARTESIAN_POINT('Ctrl Pts',(0.396862696659689,0.05,-1.50628520096425));
#8231=CARTESIAN_POINT('Ctrl Pts',(0.396862696659689,0.05,-1.5));
#8232=CARTESIAN_POINT('',(1.2,-6.12323399573677E-18,-1.45));
#8233=CARTESIAN_POINT('',(-1.3,-6.12323399573677E-18,-1.45));
#8234=CARTESIAN_POINT('',(1.19895788082818,0.05,-1.5));
#8235=CARTESIAN_POINT('Ctrl Pts',(1.19895788082818,0.05,-1.5));
#8236=CARTESIAN_POINT('Ctrl Pts',(1.19895788082818,0.05,-1.50627889147831));
#8237=CARTESIAN_POINT('Ctrl Pts',(1.19901227819454,0.0487450133099081,-1.51297580462407));
#8238=CARTESIAN_POINT('Ctrl Pts',(1.19920885850753,0.0436421041657013,-1.52529455629072));
#8239=CARTESIAN_POINT('Ctrl Pts',(1.1993482149535,0.0397942217705328,-1.53091645634812));
#8240=CARTESIAN_POINT('Ctrl Pts',(1.19960989221221,0.0309164568000038,-1.53979422131865));
#8241=CARTESIAN_POINT('Ctrl Pts',(1.19974919586288,0.0252945565319674,-1.54364210404195));
#8242=CARTESIAN_POINT('Ctrl Pts',(1.19994565546462,0.0129758042228729,-1.54874501349991));
#8243=CARTESIAN_POINT('Ctrl Pts',(1.2,0.00627889083911038,-1.55));
#8244=CARTESIAN_POINT('Ctrl Pts',(1.2,-0.00627889083911041,-1.55));
#8245=CARTESIAN_POINT('Ctrl Pts',(1.19994565546462,-0.0129758042228729,
-1.54874501349991));
#8246=CARTESIAN_POINT('Ctrl Pts',(1.19974919586288,-0.0252945565319674,
-1.54364210404195));
#8247=CARTESIAN_POINT('Ctrl Pts',(1.19960989221221,-0.0309164568000038,
-1.53979422131865));
#8248=CARTESIAN_POINT('Ctrl Pts',(1.1993482149535,-0.0397942217705328,-1.53091645634812));
#8249=CARTESIAN_POINT('Ctrl Pts',(1.19920885850753,-0.0436421041657012,
-1.52529455629072));
#8250=CARTESIAN_POINT('Ctrl Pts',(1.19901227819454,-0.0487450133099081,
-1.51297580462407));
#8251=CARTESIAN_POINT('Ctrl Pts',(1.19895788082818,-0.05,-1.50627889147831));
#8252=CARTESIAN_POINT('Ctrl Pts',(1.19895788082818,-0.05,-1.49372110852169));
#8253=CARTESIAN_POINT('Ctrl Pts',(1.19901227819454,-0.0487450133099082,
-1.48702419537594));
#8254=CARTESIAN_POINT('Ctrl Pts',(1.19920885850753,-0.0436421041657014,
-1.47470544370928));
#8255=CARTESIAN_POINT('Ctrl Pts',(1.1993482149535,-0.0397942217705328,-1.46908354365188));
#8256=CARTESIAN_POINT('Ctrl Pts',(1.19960989221221,-0.0309164568000038,
-1.46020577868135));
#8257=CARTESIAN_POINT('Ctrl Pts',(1.19974919586288,-0.0252945565319675,
-1.45635789595805));
#8258=CARTESIAN_POINT('Ctrl Pts',(1.19994565546462,-0.0129758042228731,
-1.45125498650009));
#8259=CARTESIAN_POINT('Ctrl Pts',(1.2,-0.00627889083911039,-1.45));
#8260=CARTESIAN_POINT('Ctrl Pts',(1.2,9.10729824887824E-18,-1.45));
#8261=CARTESIAN_POINT('Ctrl Pts',(1.2,9.10729824887039E-18,-1.45));
#8262=CARTESIAN_POINT('Ctrl Pts',(1.2,0.00627889083911039,-1.45));
#8263=CARTESIAN_POINT('Ctrl Pts',(1.19994565546462,0.012975804222873,-1.45125498650009));
#8264=CARTESIAN_POINT('Ctrl Pts',(1.19974919586288,0.0252945565319674,-1.45635789595805));
#8265=CARTESIAN_POINT('Ctrl Pts',(1.19960989221221,0.0309164568000038,-1.46020577868135));
#8266=CARTESIAN_POINT('Ctrl Pts',(1.1993482149535,0.0397942217705329,-1.46908354365188));
#8267=CARTESIAN_POINT('Ctrl Pts',(1.19920885850753,0.0436421041657014,-1.47470544370928));
#8268=CARTESIAN_POINT('Ctrl Pts',(1.19901227819454,0.0487450133099082,-1.48702419537594));
#8269=CARTESIAN_POINT('Ctrl Pts',(1.19895788082818,0.05,-1.49372110852169));
#8270=CARTESIAN_POINT('Ctrl Pts',(1.19895788082818,0.05,-1.5));
#8271=CARTESIAN_POINT('Origin',(-1.3,0.,-0.5));
#8272=CARTESIAN_POINT('',(-1.19895788082818,0.05,-0.5));
#8273=CARTESIAN_POINT('',(-1.2,-6.12323399573677E-18,-0.45));
#8274=CARTESIAN_POINT('Ctrl Pts',(-1.19895788082818,0.05,-0.5));
#8275=CARTESIAN_POINT('Ctrl Pts',(-1.19895788082818,0.05,-0.493721108521693));
#8276=CARTESIAN_POINT('Ctrl Pts',(-1.19901227819454,0.0487450133099082,
-0.487024195375935));
#8277=CARTESIAN_POINT('Ctrl Pts',(-1.19920885850753,0.0436421041657014,
-0.47470544370928));
#8278=CARTESIAN_POINT('Ctrl Pts',(-1.1993482149535,0.0397942217705329,-0.469083543651878));
#8279=CARTESIAN_POINT('Ctrl Pts',(-1.19960989221221,0.0309164568000038,
-0.460205778681349));
#8280=CARTESIAN_POINT('Ctrl Pts',(-1.19974919586288,0.0252945565319675,
-0.456357895958046));
#8281=CARTESIAN_POINT('Ctrl Pts',(-1.19994565546462,0.012975804222873,-0.451254986500089));
#8282=CARTESIAN_POINT('Ctrl Pts',(-1.2,0.00627889083911039,-0.45));
#8283=CARTESIAN_POINT('Ctrl Pts',(-1.2,7.37257477290143E-18,-0.45));
#8284=CARTESIAN_POINT('',(-1.2,-8.08513827217387E-17,-0.55));
#8285=CARTESIAN_POINT('Ctrl Pts',(-1.2,-1.47451495458029E-17,-0.55));
#8286=CARTESIAN_POINT('Ctrl Pts',(-1.2,0.0062788908391104,-0.55));
#8287=CARTESIAN_POINT('Ctrl Pts',(-1.19994565546462,0.0129758042228731,
-0.548745013499911));
#8288=CARTESIAN_POINT('Ctrl Pts',(-1.19974919586288,0.0252945565319676,
-0.543642104041954));
#8289=CARTESIAN_POINT('Ctrl Pts',(-1.19960989221221,0.0309164568000038,
-0.539794221318651));
#8290=CARTESIAN_POINT('Ctrl Pts',(-1.1993482149535,0.0397942217705328,-0.530916456348121));
#8291=CARTESIAN_POINT('Ctrl Pts',(-1.19920885850753,0.0436421041657015,
-0.52529455629072));
#8292=CARTESIAN_POINT('Ctrl Pts',(-1.19901227819454,0.0487450133099082,
-0.512975804624065));
#8293=CARTESIAN_POINT('Ctrl Pts',(-1.19895788082818,0.05,-0.506278891478307));
#8294=CARTESIAN_POINT('Ctrl Pts',(-1.19895788082818,0.05,-0.5));
#8295=CARTESIAN_POINT('Ctrl Pts',(-1.2,7.37257477290143E-18,-0.45));
#8296=CARTESIAN_POINT('Ctrl Pts',(-1.2,-0.00627889083911038,-0.45));
#8297=CARTESIAN_POINT('Ctrl Pts',(-1.19994565546462,-0.012975804222873,
-0.451254986500089));
#8298=CARTESIAN_POINT('Ctrl Pts',(-1.19974919586288,-0.0252945565319675,
-0.456357895958046));
#8299=CARTESIAN_POINT('Ctrl Pts',(-1.19960989221221,-0.0309164568000038,
-0.460205778681349));
#8300=CARTESIAN_POINT('Ctrl Pts',(-1.1993482149535,-0.0397942217705328,
-0.469083543651878));
#8301=CARTESIAN_POINT('Ctrl Pts',(-1.19920885850753,-0.0436421041657014,
-0.47470544370928));
#8302=CARTESIAN_POINT('Ctrl Pts',(-1.19901227819454,-0.0487450133099082,
-0.487024195375935));
#8303=CARTESIAN_POINT('Ctrl Pts',(-1.19895788082818,-0.05,-0.493721108521693));
#8304=CARTESIAN_POINT('Ctrl Pts',(-1.19895788082818,-0.05,-0.506278891478307));
#8305=CARTESIAN_POINT('Ctrl Pts',(-1.19901227819454,-0.0487450133099082,
-0.512975804624065));
#8306=CARTESIAN_POINT('Ctrl Pts',(-1.19920885850753,-0.0436421041657015,
-0.52529455629072));
#8307=CARTESIAN_POINT('Ctrl Pts',(-1.1993482149535,-0.0397942217705328,
-0.530916456348121));
#8308=CARTESIAN_POINT('Ctrl Pts',(-1.19960989221221,-0.0309164568000039,
-0.539794221318651));
#8309=CARTESIAN_POINT('Ctrl Pts',(-1.19974919586288,-0.0252945565319676,
-0.543642104041954));
#8310=CARTESIAN_POINT('Ctrl Pts',(-1.19994565546462,-0.0129758042228732,
-0.548745013499911));
#8311=CARTESIAN_POINT('Ctrl Pts',(-1.2,-0.00627889083911043,-0.55));
#8312=CARTESIAN_POINT('Ctrl Pts',(-1.2,-1.4745149545795E-17,-0.55));
#8313=CARTESIAN_POINT('',(-0.4,-6.0973830808278E-18,-0.45));
#8314=CARTESIAN_POINT('',(-1.3,-6.12323399573677E-18,-0.45));
#8315=CARTESIAN_POINT('',(-0.4,-2.44929359829471E-17,-0.55));
#8316=CARTESIAN_POINT('Ctrl Pts',(-0.4,0.,-0.55));
#8317=CARTESIAN_POINT('Ctrl Pts',(-0.4,-0.00628514845714647,-0.55));
#8318=CARTESIAN_POINT('Ctrl Pts',(-0.399836729543542,-0.0129847676279313,
-0.548742566758595));
#8319=CARTESIAN_POINT('Ctrl Pts',(-0.399246581249293,-0.0253018150396576,
-0.543637829363298));
#8320=CARTESIAN_POINT('Ctrl Pts',(-0.398828027526425,-0.0309197907817458,
-0.539790887336909));
#8321=CARTESIAN_POINT('Ctrl Pts',(-0.398040841710914,-0.0397909243921697,
-0.530919753726485));
#8322=CARTESIAN_POINT('Ctrl Pts',(-0.397620851691571,-0.0436378373878619,
-0.525301794093861));
#8323=CARTESIAN_POINT('Ctrl Pts',(-0.397027412247524,-0.0487425534891115,
-0.512984801229014));
#8324=CARTESIAN_POINT('Ctrl Pts',(-0.396862696659689,-0.05,-0.506285200964255));
#8325=CARTESIAN_POINT('Ctrl Pts',(-0.396862696659689,-0.05,-0.493714799035745));
#8326=CARTESIAN_POINT('Ctrl Pts',(-0.397027412247524,-0.0487425534891115,
-0.487015198770986));
#8327=CARTESIAN_POINT('Ctrl Pts',(-0.397620851691571,-0.0436378373878619,
-0.474698205906139));
#8328=CARTESIAN_POINT('Ctrl Pts',(-0.398040841710914,-0.0397909243921697,
-0.469080246273515));
#8329=CARTESIAN_POINT('Ctrl Pts',(-0.398828027526425,-0.0309197907817458,
-0.460209112663091));
#8330=CARTESIAN_POINT('Ctrl Pts',(-0.399246581249293,-0.0253018150396576,
-0.456362170636702));
#8331=CARTESIAN_POINT('Ctrl Pts',(-0.399836729543542,-0.0129847676279313,
-0.451257433241405));
#8332=CARTESIAN_POINT('Ctrl Pts',(-0.4,-0.00628514845714648,-0.45));
#8333=CARTESIAN_POINT('Ctrl Pts',(-0.4,-6.07153216591882E-18,-0.45));
#8334=CARTESIAN_POINT('',(-0.396862696659689,0.05,-0.5));
#8335=CARTESIAN_POINT('Ctrl Pts',(-0.396862696659689,0.05,-0.5));
#8336=CARTESIAN_POINT('Ctrl Pts',(-0.396862696659689,0.05,-0.506285200964255));
#8337=CARTESIAN_POINT('Ctrl Pts',(-0.397027412247524,0.0487425534891115,
-0.512984801229014));
#8338=CARTESIAN_POINT('Ctrl Pts',(-0.397620851691571,0.0436378373878619,
-0.525301794093861));
#8339=CARTESIAN_POINT('Ctrl Pts',(-0.398040841710914,0.0397909243921697,
-0.530919753726485));
#8340=CARTESIAN_POINT('Ctrl Pts',(-0.398828027526425,0.0309197907817458,
-0.539790887336909));
#8341=CARTESIAN_POINT('Ctrl Pts',(-0.399246581249293,0.0253018150396576,
-0.543637829363298));
#8342=CARTESIAN_POINT('Ctrl Pts',(-0.399836729543542,0.0129847676279313,
-0.548742566758595));
#8343=CARTESIAN_POINT('Ctrl Pts',(-0.4,0.00628514845714647,-0.55));
#8344=CARTESIAN_POINT('Ctrl Pts',(-0.4,0.,-0.55));
#8345=CARTESIAN_POINT('Ctrl Pts',(-0.4,-6.07153216591882E-18,-0.45));
#8346=CARTESIAN_POINT('Ctrl Pts',(-0.4,0.00628514845714647,-0.45));
#8347=CARTESIAN_POINT('Ctrl Pts',(-0.399836729543542,0.0129847676279313,
-0.451257433241405));
#8348=CARTESIAN_POINT('Ctrl Pts',(-0.399246581249293,0.0253018150396577,
-0.456362170636702));
#8349=CARTESIAN_POINT('Ctrl Pts',(-0.398828027526425,0.0309197907817458,
-0.460209112663091));
#8350=CARTESIAN_POINT('Ctrl Pts',(-0.398040841710914,0.0397909243921697,
-0.469080246273515));
#8351=CARTESIAN_POINT('Ctrl Pts',(-0.397620851691571,0.0436378373878619,
-0.474698205906139));
#8352=CARTESIAN_POINT('Ctrl Pts',(-0.397027412247524,0.0487425534891115,
-0.487015198770986));
#8353=CARTESIAN_POINT('Ctrl Pts',(-0.396862696659689,0.05,-0.493714799035745));
#8354=CARTESIAN_POINT('Ctrl Pts',(-0.396862696659689,0.05,-0.5));
#8355=CARTESIAN_POINT('Origin',(-1.3,0.,-0.5));
#8356=CARTESIAN_POINT('',(0.396862696659689,0.05,-0.5));
#8357=CARTESIAN_POINT('',(0.4,-6.3142235153249E-18,-0.45));
#8358=CARTESIAN_POINT('Ctrl Pts',(0.396862696659689,0.05,-0.5));
#8359=CARTESIAN_POINT('Ctrl Pts',(0.396862696659689,0.05,-0.493714799035745));
#8360=CARTESIAN_POINT('Ctrl Pts',(0.397027412247524,0.0487425534891115,
-0.487015198770986));
#8361=CARTESIAN_POINT('Ctrl Pts',(0.397620851691571,0.0436378373878619,
-0.474698205906139));
#8362=CARTESIAN_POINT('Ctrl Pts',(0.398040841710914,0.0397909243921697,
-0.469080246273515));
#8363=CARTESIAN_POINT('Ctrl Pts',(0.398828027526425,0.0309197907817458,
-0.460209112663091));
#8364=CARTESIAN_POINT('Ctrl Pts',(0.399246581249293,0.0253018150396576,
-0.456362170636702));
#8365=CARTESIAN_POINT('Ctrl Pts',(0.399836729543542,0.0129847676279312,
-0.451257433241405));
#8366=CARTESIAN_POINT('Ctrl Pts',(0.4,0.00628514845714647,-0.45));
#8367=CARTESIAN_POINT('Ctrl Pts',(0.4,-6.50521303491303E-18,-0.45));
#8368=CARTESIAN_POINT('Ctrl Pts',(0.4,-6.50521303491303E-18,-0.45));
#8369=CARTESIAN_POINT('Ctrl Pts',(0.4,-0.00628514845714648,-0.45));
#8370=CARTESIAN_POINT('Ctrl Pts',(0.399836729543542,-0.0129847676279313,
-0.451257433241405));
#8371=CARTESIAN_POINT('Ctrl Pts',(0.399246581249293,-0.0253018150396576,
-0.456362170636702));
#8372=CARTESIAN_POINT('Ctrl Pts',(0.398828027526425,-0.0309197907817458,
-0.460209112663091));
#8373=CARTESIAN_POINT('Ctrl Pts',(0.398040841710914,-0.0397909243921697,
-0.469080246273515));
#8374=CARTESIAN_POINT('Ctrl Pts',(0.397620851691571,-0.0436378373878619,
-0.474698205906139));
#8375=CARTESIAN_POINT('Ctrl Pts',(0.397027412247524,-0.0487425534891115,
-0.487015198770986));
#8376=CARTESIAN_POINT('Ctrl Pts',(0.396862696659689,-0.05,-0.493714799035745));
#8377=CARTESIAN_POINT('Ctrl Pts',(0.396862696659689,-0.05,-0.506285200964255));
#8378=CARTESIAN_POINT('Ctrl Pts',(0.397027412247524,-0.0487425534891115,
-0.512984801229014));
#8379=CARTESIAN_POINT('Ctrl Pts',(0.397620851691571,-0.0436378373878619,
-0.525301794093861));
#8380=CARTESIAN_POINT('Ctrl Pts',(0.398040841710914,-0.0397909243921697,
-0.530919753726485));
#8381=CARTESIAN_POINT('Ctrl Pts',(0.398828027526425,-0.0309197907817458,
-0.539790887336909));
#8382=CARTESIAN_POINT('Ctrl Pts',(0.399246581249293,-0.0253018150396576,
-0.543637829363298));
#8383=CARTESIAN_POINT('Ctrl Pts',(0.399836729543542,-0.0129847676279313,
-0.548742566758595));
#8384=CARTESIAN_POINT('Ctrl Pts',(0.4,-0.00628514845714647,-0.55));
#8385=CARTESIAN_POINT('Ctrl Pts',(0.4,0.00628514845714647,-0.55));
#8386=CARTESIAN_POINT('Ctrl Pts',(0.399836729543542,0.0129847676279313,
-0.548742566758595));
#8387=CARTESIAN_POINT('Ctrl Pts',(0.399246581249293,0.0253018150396576,
-0.543637829363298));
#8388=CARTESIAN_POINT('Ctrl Pts',(0.398828027526425,0.0309197907817458,
-0.539790887336909));
#8389=CARTESIAN_POINT('Ctrl Pts',(0.398040841710914,0.0397909243921697,
-0.530919753726485));
#8390=CARTESIAN_POINT('Ctrl Pts',(0.397620851691571,0.043637837387862,-0.525301794093861));
#8391=CARTESIAN_POINT('Ctrl Pts',(0.397027412247524,0.0487425534891116,
-0.512984801229014));
#8392=CARTESIAN_POINT('Ctrl Pts',(0.396862696659689,0.05,-0.506285200964255));
#8393=CARTESIAN_POINT('Ctrl Pts',(0.396862696659689,0.05,-0.5));
#8394=CARTESIAN_POINT('',(1.2,-6.12323399573677E-18,-0.45));
#8395=CARTESIAN_POINT('',(-1.3,-6.12323399573677E-18,-0.45));
#8396=CARTESIAN_POINT('',(1.19895788082818,0.05,-0.5));
#8397=CARTESIAN_POINT('Ctrl Pts',(1.19895788082818,0.05,-0.5));
#8398=CARTESIAN_POINT('Ctrl Pts',(1.19895788082818,0.05,-0.506278891478307));
#8399=CARTESIAN_POINT('Ctrl Pts',(1.19901227819454,0.0487450133099082,-0.512975804624065));
#8400=CARTESIAN_POINT('Ctrl Pts',(1.19920885850753,0.0436421041657015,-0.52529455629072));
#8401=CARTESIAN_POINT('Ctrl Pts',(1.1993482149535,0.0397942217705328,-0.530916456348121));
#8402=CARTESIAN_POINT('Ctrl Pts',(1.19960989221221,0.0309164568000038,-0.539794221318651));
#8403=CARTESIAN_POINT('Ctrl Pts',(1.19974919586288,0.0252945565319676,-0.543642104041954));
#8404=CARTESIAN_POINT('Ctrl Pts',(1.19994565546462,0.0129758042228732,-0.548745013499911));
#8405=CARTESIAN_POINT('Ctrl Pts',(1.2,0.00627889083911041,-0.55));
#8406=CARTESIAN_POINT('Ctrl Pts',(1.2,-0.00627889083911043,-0.55));
#8407=CARTESIAN_POINT('Ctrl Pts',(1.19994565546462,-0.0129758042228732,
-0.548745013499911));
#8408=CARTESIAN_POINT('Ctrl Pts',(1.19974919586288,-0.0252945565319676,
-0.543642104041954));
#8409=CARTESIAN_POINT('Ctrl Pts',(1.19960989221221,-0.0309164568000039,
-0.539794221318651));
#8410=CARTESIAN_POINT('Ctrl Pts',(1.1993482149535,-0.0397942217705328,-0.530916456348121));
#8411=CARTESIAN_POINT('Ctrl Pts',(1.19920885850753,-0.0436421041657015,
-0.52529455629072));
#8412=CARTESIAN_POINT('Ctrl Pts',(1.19901227819454,-0.0487450133099082,
-0.512975804624065));
#8413=CARTESIAN_POINT('Ctrl Pts',(1.19895788082818,-0.05,-0.506278891478307));
#8414=CARTESIAN_POINT('Ctrl Pts',(1.19895788082818,-0.05,-0.493721108521693));
#8415=CARTESIAN_POINT('Ctrl Pts',(1.19901227819454,-0.0487450133099082,
-0.487024195375935));
#8416=CARTESIAN_POINT('Ctrl Pts',(1.19920885850753,-0.0436421041657014,
-0.47470544370928));
#8417=CARTESIAN_POINT('Ctrl Pts',(1.1993482149535,-0.0397942217705328,-0.469083543651878));
#8418=CARTESIAN_POINT('Ctrl Pts',(1.19960989221221,-0.0309164568000038,
-0.460205778681349));
#8419=CARTESIAN_POINT('Ctrl Pts',(1.19974919586288,-0.0252945565319675,
-0.456357895958046));
#8420=CARTESIAN_POINT('Ctrl Pts',(1.19994565546462,-0.012975804222873,-0.451254986500089));
#8421=CARTESIAN_POINT('Ctrl Pts',(1.2,-0.00627889083911039,-0.45));
#8422=CARTESIAN_POINT('Ctrl Pts',(1.2,3.90312782094782E-18,-0.45));
#8423=CARTESIAN_POINT('Ctrl Pts',(1.2,3.90312782093996E-18,-0.45));
#8424=CARTESIAN_POINT('Ctrl Pts',(1.2,0.00627889083911039,-0.45));
#8425=CARTESIAN_POINT('Ctrl Pts',(1.19994565546462,0.012975804222873,-0.451254986500089));
#8426=CARTESIAN_POINT('Ctrl Pts',(1.19974919586288,0.0252945565319675,-0.456357895958046));
#8427=CARTESIAN_POINT('Ctrl Pts',(1.19960989221221,0.0309164568000038,-0.460205778681349));
#8428=CARTESIAN_POINT('Ctrl Pts',(1.1993482149535,0.0397942217705329,-0.469083543651878));
#8429=CARTESIAN_POINT('Ctrl Pts',(1.19920885850753,0.0436421041657014,-0.47470544370928));
#8430=CARTESIAN_POINT('Ctrl Pts',(1.19901227819454,0.0487450133099082,-0.487024195375935));
#8431=CARTESIAN_POINT('Ctrl Pts',(1.19895788082818,0.05,-0.493721108521693));
#8432=CARTESIAN_POINT('Ctrl Pts',(1.19895788082818,0.05,-0.5));
#8433=CARTESIAN_POINT('Origin',(0.,0.,-3.2));
#8434=CARTESIAN_POINT('',(-0.4,-4.89858719658941E-17,-3.2));
#8435=CARTESIAN_POINT('Origin',(0.,0.,-3.2));
#8436=CARTESIAN_POINT('',(-0.4,-4.89858719658941E-17,-3.2));
#8437=CARTESIAN_POINT('',(-0.4,-4.89858719658941E-17,-3.2));
#8438=CARTESIAN_POINT('',(-0.4,-4.89858719658941E-17,-3.2));
#8439=CARTESIAN_POINT('',(-0.4,4.89858719658941E-17,1.4));
#8440=CARTESIAN_POINT('',(-0.4,-4.89858719658941E-17,-3.2));
#8441=CARTESIAN_POINT('Origin',(0.,0.,1.4));
#8442=CARTESIAN_POINT('Origin',(0.,0.,-3.2));
#8443=CARTESIAN_POINT('Origin',(0.,0.,-0.3));
#8444=CARTESIAN_POINT('',(-0.6185,-7.57444045272638E-17,1.4));
#8445=CARTESIAN_POINT('Origin',(0.,0.,1.4));
#8446=CARTESIAN_POINT('',(-0.6185,-7.57444045272638E-17,-0.3));
#8447=CARTESIAN_POINT('',(-0.6185,-7.57444045272638E-17,-0.3));
#8448=CARTESIAN_POINT('Origin',(0.,0.,-0.3));
#8449=CARTESIAN_POINT('Origin',(0.,0.,1.4));
#8450=CARTESIAN_POINT('Origin',(0.,0.,-3.5));
#8451=CARTESIAN_POINT('',(-1.2,-1.46957615897682E-16,-0.3));
#8452=CARTESIAN_POINT('Origin',(0.,0.,-0.3));
#8453=CARTESIAN_POINT('',(-1.2,-1.46957615897682E-16,-3.5));
#8454=CARTESIAN_POINT('',(-1.2,-1.46957615897682E-16,-3.5));
#8455=CARTESIAN_POINT('',(-1.2,-1.46957615897682E-16,-3.5));
#8456=CARTESIAN_POINT('',(-1.2,-1.46957615897682E-16,-3.5));
#8457=CARTESIAN_POINT('',(-1.2,-1.46957615897682E-16,-3.5));
#8458=CARTESIAN_POINT('Origin',(0.,0.,-3.5));
#8459=CARTESIAN_POINT('Origin',(0.,0.,-0.3));
#8460=CARTESIAN_POINT('Origin',(0.,0.,-3.5));
#10220=UNCERTAINTY_MEASURE_WITH_UNIT(LENGTH_MEASURE(0.001),#10267,
'DISTANCE_ACCURACY_VALUE',
'Maximum model space distance between geometric entities at asserted c
onnectivities');
#10241=UNCERTAINTY_MEASURE_WITH_UNIT(LENGTH_MEASURE(0.001),#10267,
'DISTANCE_ACCURACY_VALUE',
'Maximum model space distance between geometric entities at asserted c
onnectivities');
#10245=(
GEOMETRIC_REPRESENTATION_CONTEXT(3)
GLOBAL_UNCERTAINTY_ASSIGNED_CONTEXT((#10220))
GLOBAL_UNIT_ASSIGNED_CONTEXT((#10267,#10269,#10270))
REPRESENTATION_CONTEXT('','3D')
);
#10266=(
GEOMETRIC_REPRESENTATION_CONTEXT(3)
GLOBAL_UNCERTAINTY_ASSIGNED_CONTEXT((#10241))
GLOBAL_UNIT_ASSIGNED_CONTEXT((#10267,#10269,#10270))
REPRESENTATION_CONTEXT('','3D')
);
#10267=(
LENGTH_UNIT()
NAMED_UNIT(*)
SI_UNIT(.CENTI.,.METRE.)
);
#10269=(
NAMED_UNIT(*)
PLANE_ANGLE_UNIT()
SI_UNIT($,.RADIAN.)
);
#10270=(
NAMED_UNIT(*)
SI_UNIT($,.STERADIAN.)
SOLID_ANGLE_UNIT()
);
#10274=SHAPE_DEFINITION_REPRESENTATION(#10298,#10357);
#10298=PRODUCT_DEFINITION_SHAPE('',$,#10382);
#10357=SHAPE_REPRESENTATION('',(#5118),#10245);
#10378=PRODUCT_DEFINITION_CONTEXT('part definition',#10452,'design');
#10382=PRODUCT_DEFINITION('Perforated filter insert',
'Perforated filter insert',#10406,#10378);
#10406=PRODUCT_DEFINITION_FORMATION('',$,#10457);
#10452=APPLICATION_CONTEXT(
'Core Data for Automotive Mechanical Design Process');
#10453=PRODUCT_CONTEXT('part definition',#10452,'mechanical');
#10457=PRODUCT('Perforated filter insert','Perforated filter insert',
'Perforated filter insert',(#10453));
#10555=COLOUR_RGB('Off White',0.89,0.88,0.83);
#10556=FILL_AREA_STYLE_COLOUR('',#10555);
#10557=FILL_AREA_STYLE('',(#10556));
#10558=SURFACE_STYLE_FILL_AREA(#10557);
#10559=SURFACE_SIDE_STYLE('',(#10558));
#10560=SURFACE_STYLE_USAGE(.BOTH.,#10559);
#10561=PRESENTATION_STYLE_ASSIGNMENT((#10560));
ENDSEC;
END-ISO-10303-21;
